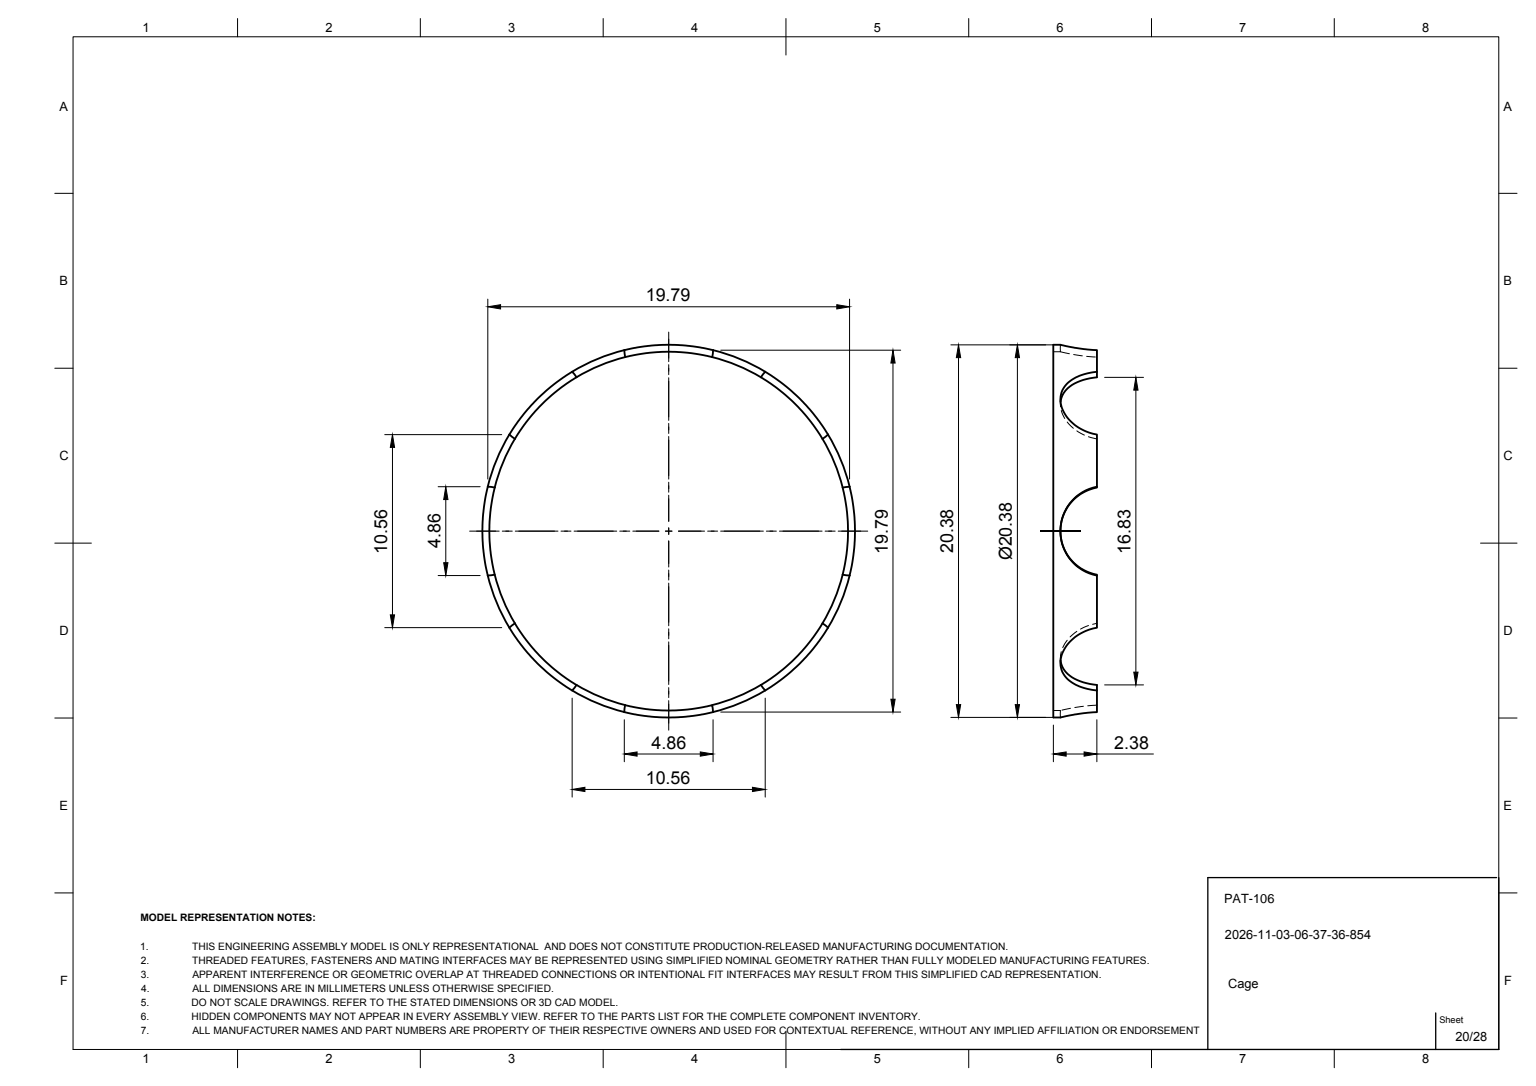
ISO-10303-21;
HEADER;
/* Generated by software containing ST-Developer
 * from STEP Tools, Inc. (www.steptools.com) 
 */

FILE_DESCRIPTION(
/* description */ ('Torsion-spring ratchet demonstrator'),
/* implementation_level */ '2;1');

FILE_NAME(
/* name */ 'Cage.step',
/* time_stamp */ '2026-10-29T17:29:17-07:00',
/* author */ (''),
/* organization */ (''),
/* preprocessor_version */ 'ST-DEVELOPER v20.2',
/* originating_system */ 'Autodesk Translation Framework v15.17.0.0',
/* authorisation */ '');

FILE_SCHEMA (('AUTOMOTIVE_DESIGN { 1 0 10303 214 3 1 1 }'));
ENDSEC;

DATA;
#10=MECHANICAL_DESIGN_GEOMETRIC_PRESENTATION_REPRESENTATION('',(#302),#11258);
#178=SPHERICAL_SURFACE('',#5739,0.247676);
#179=SPHERICAL_SURFACE('',#5755,0.247676);
#180=SPHERICAL_SURFACE('',#5760,0.247676);
#181=SPHERICAL_SURFACE('',#5765,0.247676);
#182=SPHERICAL_SURFACE('',#5770,0.247676);
#183=SPHERICAL_SURFACE('',#5775,0.247676);
#184=SPHERICAL_SURFACE('',#5780,0.247676);
#185=SPHERICAL_SURFACE('',#5788,0.247676);
#205=B_SPLINE_CURVE_WITH_KNOTS('',3,(#8316,#8317,#8318,#8319,#8320,#8321,
#8322,#8323,#8324,#8325,#8326,#8327,#8328,#8329,#8330,#8331,#8332,#8333,
#8334,#8335,#8336,#8337),.UNSPECIFIED.,.F.,.F.,(4,2,2,2,2,2,2,2,2,2,4),
(0.0473477652366656,0.126350602536658,0.189525903804987,0.252701205073317,
0.313298422430275,0.373895639787233,0.434492857144191,0.495090074501149,
0.558265375769478,0.621440677037807,0.7004435143378),.UNSPECIFIED.);
#206=B_SPLINE_CURVE_WITH_KNOTS('',3,(#8341,#8342,#8343,#8344,#8345,#8346,
#8347,#8348,#8349,#8350,#8351,#8352,#8353,#8354,#8355,#8356,#8357,#8358,
#8359,#8360,#8361,#8362),.UNSPECIFIED.,.F.,.F.,(4,2,2,2,2,2,2,2,2,2,4),
(0.0464897534940957,0.0852567806515119,0.170513561303024,0.246687263103517,
0.308657850341199,0.370628437578881,0.432599024816563,0.494569612054245,
0.570743313854739,0.656000094506251,0.694767121663666),.UNSPECIFIED.);
#207=B_SPLINE_CURVE_WITH_KNOTS('',3,(#8368,#8369,#8370,#8371,#8372,#8373,
#8374,#8375,#8376,#8377,#8378,#8379,#8380,#8381,#8382,#8383,#8384,#8385,
#8386,#8387,#8388,#8389),.UNSPECIFIED.,.F.,.F.,(4,2,2,2,2,2,2,2,2,2,4),
(0.0464897534940957,0.0852567806515118,0.170513561303024,0.246687263103517,
0.308657850341199,0.370628437578881,0.432599024816563,0.494569612054245,
0.570743313854738,0.65600009450625,0.694767121663666),.UNSPECIFIED.);
#208=B_SPLINE_CURVE_WITH_KNOTS('',3,(#8393,#8394,#8395,#8396,#8397,#8398,
#8399,#8400,#8401,#8402,#8403,#8404,#8405,#8406,#8407,#8408,#8409,#8410,
#8411,#8412,#8413,#8414),.UNSPECIFIED.,.F.,.F.,(4,2,2,2,2,2,2,2,2,2,4),
(0.0464897534940957,0.0852567806515119,0.170513561303024,0.246687263103517,
0.308657850341199,0.370628437578881,0.432599024816563,0.494569612054245,
0.570743313854739,0.656000094506251,0.694767121663666),.UNSPECIFIED.);
#209=B_SPLINE_CURVE_WITH_KNOTS('',3,(#8418,#8419,#8420,#8421,#8422,#8423,
#8424,#8425,#8426,#8427,#8428,#8429),.UNSPECIFIED.,.F.,.F.,(4,2,2,2,2,4),
(0.0464897534940957,0.0852567806515119,0.170513561303024,0.246687263103517,
0.308657850341199,0.370628437578881),.UNSPECIFIED.);
#210=B_SPLINE_CURVE_WITH_KNOTS('',3,(#8434,#8435,#8436,#8437,#8438,#8439,
#8440,#8441,#8442,#8443,#8444,#8445),.UNSPECIFIED.,.F.,.F.,(4,2,2,2,2,4),
(0.370628437578881,0.432599024816563,0.494569612054245,0.570743313854738,
0.65600009450625,0.694767121663666),.UNSPECIFIED.);
#211=B_SPLINE_CURVE_WITH_KNOTS('',3,(#8449,#8450,#8451,#8452,#8453,#8454,
#8455,#8456,#8457,#8458,#8459,#8460,#8461,#8462,#8463,#8464,#8465,#8466,
#8467,#8468,#8469,#8470),.UNSPECIFIED.,.F.,.F.,(4,2,2,2,2,2,2,2,2,2,4),
(0.0464897534940957,0.0852567806515121,0.170513561303024,0.246687263103518,
0.308657850341199,0.370628437578881,0.432599024816563,0.494569612054245,
0.570743313854738,0.65600009450625,0.694767121663666),.UNSPECIFIED.);
#212=B_SPLINE_CURVE_WITH_KNOTS('',3,(#8474,#8475,#8476,#8477,#8478,#8479,
#8480,#8481,#8482,#8483,#8484,#8485,#8486,#8487,#8488,#8489,#8490,#8491,
#8492,#8493,#8494,#8495),.UNSPECIFIED.,.F.,.F.,(4,2,2,2,2,2,2,2,2,2,4),
(0.0464897534940957,0.0852567806515119,0.170513561303024,0.246687263103517,
0.308657850341199,0.370628437578881,0.432599024816563,0.494569612054245,
0.570743313854738,0.65600009450625,0.694767121663667),.UNSPECIFIED.);
#213=B_SPLINE_CURVE_WITH_KNOTS('',3,(#8499,#8500,#8501,#8502,#8503,#8504,
#8505,#8506,#8507,#8508,#8509,#8510,#8511,#8512,#8513,#8514,#8515,#8516,
#8517,#8518,#8519,#8520),.UNSPECIFIED.,.F.,.F.,(4,2,2,2,2,2,2,2,2,2,4),
(0.0464897534940957,0.0852567806515119,0.170513561303024,0.246687263103517,
0.308657850341199,0.370628437578881,0.432599024816563,0.494569612054245,
0.570743313854738,0.65600009450625,0.694767121663666),.UNSPECIFIED.);
#214=B_SPLINE_CURVE_WITH_KNOTS('',3,(#8524,#8525,#8526,#8527,#8528,#8529,
#8530,#8531,#8532,#8533,#8534,#8535,#8536,#8537,#8538,#8539,#8540,#8541,
#8542,#8543,#8544,#8545),.UNSPECIFIED.,.F.,.F.,(4,2,2,2,2,2,2,2,2,2,4),
(0.0464897534940957,0.0852567806515119,0.170513561303024,0.246687263103517,
0.308657850341199,0.370628437578881,0.432599024816563,0.494569612054245,
0.570743313854739,0.656000094506251,0.694767121663667),.UNSPECIFIED.);
#215=B_SPLINE_CURVE_WITH_KNOTS('',3,(#8553,#8554,#8555,#8556,#8557,#8558,
#8559,#8560,#8561,#8562,#8563,#8564,#8565,#8566,#8567,#8568,#8569,#8570,
#8571,#8572,#8573,#8574),.UNSPECIFIED.,.F.,.F.,(4,2,2,2,2,2,2,2,2,2,4),
(0.0473477652366656,0.126350602536658,0.189525903804987,0.252701205073316,
0.313298422430274,0.373895639787232,0.434492857144191,0.495090074501149,
0.558265375769478,0.621440677037807,0.7004435143378),.UNSPECIFIED.);
#216=B_SPLINE_CURVE_WITH_KNOTS('',3,(#8582,#8583,#8584,#8585,#8586,#8587,
#8588,#8589,#8590,#8591,#8592,#8593,#8594,#8595,#8596,#8597,#8598,#8599,
#8600,#8601,#8602,#8603),.UNSPECIFIED.,.F.,.F.,(4,2,2,2,2,2,2,2,2,2,4),
(0.0473477652366656,0.126350602536658,0.189525903804987,0.252701205073317,
0.313298422430275,0.373895639787233,0.434492857144191,0.495090074501149,
0.558265375769478,0.621440677037807,0.7004435143378),.UNSPECIFIED.);
#217=B_SPLINE_CURVE_WITH_KNOTS('',3,(#8612,#8613,#8614,#8615,#8616,#8617,
#8618,#8619,#8620,#8621,#8622,#8623),.UNSPECIFIED.,.F.,.F.,(4,2,2,2,2,4),
(0.0473477652366656,0.126350602536658,0.189525903804987,0.252701205073316,
0.313298422430275,0.373895639787233),.UNSPECIFIED.);
#218=B_SPLINE_CURVE_WITH_KNOTS('',3,(#8625,#8626,#8627,#8628,#8629,#8630,
#8631,#8632,#8633,#8634,#8635,#8636),.UNSPECIFIED.,.F.,.F.,(4,2,2,2,2,4),
(0.373895639787233,0.434492857144191,0.495090074501149,0.558265375769478,
0.621440677037807,0.7004435143378),.UNSPECIFIED.);
#219=B_SPLINE_CURVE_WITH_KNOTS('',3,(#8643,#8644,#8645,#8646,#8647,#8648,
#8649,#8650,#8651,#8652,#8653,#8654,#8655,#8656,#8657,#8658,#8659,#8660,
#8661,#8662,#8663,#8664),.UNSPECIFIED.,.F.,.F.,(4,2,2,2,2,2,2,2,2,2,4),
(0.0473477652366656,0.126350602536658,0.189525903804987,0.252701205073316,
0.313298422430275,0.373895639787233,0.434492857144191,0.495090074501149,
0.558265375769478,0.621440677037807,0.7004435143378),.UNSPECIFIED.);
#220=B_SPLINE_CURVE_WITH_KNOTS('',3,(#8672,#8673,#8674,#8675,#8676,#8677,
#8678,#8679,#8680,#8681,#8682,#8683,#8684,#8685,#8686,#8687,#8688,#8689,
#8690,#8691,#8692,#8693),.UNSPECIFIED.,.F.,.F.,(4,2,2,2,2,2,2,2,2,2,4),
(0.0473477652366656,0.126350602536658,0.189525903804987,0.252701205073317,
0.313298422430275,0.373895639787233,0.434492857144191,0.495090074501149,
0.558265375769478,0.621440677037807,0.7004435143378),.UNSPECIFIED.);
#221=B_SPLINE_CURVE_WITH_KNOTS('',3,(#8701,#8702,#8703,#8704,#8705,#8706,
#8707,#8708,#8709,#8710,#8711,#8712,#8713,#8714,#8715,#8716,#8717,#8718,
#8719,#8720,#8721,#8722),.UNSPECIFIED.,.F.,.F.,(4,2,2,2,2,2,2,2,2,2,4),
(0.0473477652366656,0.126350602536658,0.189525903804987,0.252701205073316,
0.313298422430275,0.373895639787233,0.434492857144191,0.495090074501149,
0.558265375769478,0.621440677037807,0.7004435143378),.UNSPECIFIED.);
#222=B_SPLINE_CURVE_WITH_KNOTS('',3,(#8731,#8732,#8733,#8734,#8735,#8736,
#8737,#8738,#8739,#8740,#8741,#8742,#8743,#8744,#8745,#8746,#8747,#8748,
#8749,#8750,#8751,#8752),.UNSPECIFIED.,.F.,.F.,(4,2,2,2,2,2,2,2,2,2,4),
(0.0473477652366656,0.126350602536658,0.189525903804987,0.252701205073317,
0.313298422430275,0.373895639787233,0.434492857144191,0.495090074501149,
0.558265375769478,0.621440677037807,0.7004435143378),.UNSPECIFIED.);
#247=SHAPE_REPRESENTATION_RELATIONSHIP('SRR','None',#11374,#271);
#271=ADVANCED_BREP_SHAPE_REPRESENTATION('',(#334),#11244);
#302=STYLED_ITEM('',(#11584),#334);
#334=MANIFOLD_SOLID_BREP('Continuous crown cage',#5173);
#413=FACE_BOUND('',#1142,.T.);
#493=PLANE('',#5752);
#494=PLANE('',#5757);
#495=PLANE('',#5762);
#496=PLANE('',#5767);
#497=PLANE('',#5772);
#498=PLANE('',#5777);
#499=PLANE('',#5786);
#500=PLANE('',#5790);
#501=PLANE('',#5791);
#751=FACE_OUTER_BOUND('',#1124,.T.);
#752=FACE_OUTER_BOUND('',#1125,.T.);
#753=FACE_OUTER_BOUND('',#1126,.T.);
#754=FACE_OUTER_BOUND('',#1127,.T.);
#755=FACE_OUTER_BOUND('',#1128,.T.);
#756=FACE_OUTER_BOUND('',#1129,.T.);
#757=FACE_OUTER_BOUND('',#1130,.T.);
#758=FACE_OUTER_BOUND('',#1131,.T.);
#759=FACE_OUTER_BOUND('',#1132,.T.);
#760=FACE_OUTER_BOUND('',#1133,.T.);
#761=FACE_OUTER_BOUND('',#1134,.T.);
#762=FACE_OUTER_BOUND('',#1135,.T.);
#763=FACE_OUTER_BOUND('',#1136,.T.);
#764=FACE_OUTER_BOUND('',#1137,.T.);
#765=FACE_OUTER_BOUND('',#1138,.T.);
#766=FACE_OUTER_BOUND('',#1139,.T.);
#767=FACE_OUTER_BOUND('',#1140,.T.);
#768=FACE_OUTER_BOUND('',#1141,.T.);
#769=FACE_OUTER_BOUND('',#1143,.T.);
#1124=EDGE_LOOP('',(#3942,#3943,#3944,#3945));
#1125=EDGE_LOOP('',(#3946,#3947,#3948,#3949,#3950,#3951,#3952,#3953,#3954,
#3955,#3956,#3957,#3958,#3959,#3960,#3961,#3962,#3963,#3964,#3965));
#1126=EDGE_LOOP('',(#3966,#3967,#3968,#3969));
#1127=EDGE_LOOP('',(#3970,#3971,#3972,#3973));
#1128=EDGE_LOOP('',(#3974,#3975,#3976,#3977));
#1129=EDGE_LOOP('',(#3978,#3979,#3980,#3981));
#1130=EDGE_LOOP('',(#3982,#3983,#3984,#3985));
#1131=EDGE_LOOP('',(#3986,#3987,#3988,#3989,#3990,#3991));
#1132=EDGE_LOOP('',(#3992,#3993,#3994,#3995));
#1133=EDGE_LOOP('',(#3996,#3997,#3998,#3999));
#1134=EDGE_LOOP('',(#4000,#4001,#4002,#4003));
#1135=EDGE_LOOP('',(#4004,#4005,#4006,#4007));
#1136=EDGE_LOOP('',(#4008,#4009,#4010,#4011));
#1137=EDGE_LOOP('',(#4012,#4013,#4014,#4015));
#1138=EDGE_LOOP('',(#4016,#4017,#4018,#4019,#4020,#4021,#4022,#4023,#4024,
#4025,#4026,#4027,#4028,#4029,#4030,#4031,#4032,#4033,#4034,#4035));
#1139=EDGE_LOOP('',(#4036,#4037,#4038,#4039));
#1140=EDGE_LOOP('',(#4040,#4041,#4042,#4043));
#1141=EDGE_LOOP('',(#4044));
#1142=EDGE_LOOP('',(#4045));
#1143=EDGE_LOOP('',(#4046,#4047,#4048,#4049));
#1429=LINE('',#8431,#1812);
#1430=LINE('',#8727,#1813);
#1812=VECTOR('',#6756,1.019052);
#1813=VECTOR('',#6833,0.980948);
#2233=CIRCLE('',#5740,0.243053047864041);
#2234=CIRCLE('',#5741,0.243053047864041);
#2235=CIRCLE('',#5743,1.019052);
#2236=CIRCLE('',#5744,1.019052);
#2237=CIRCLE('',#5745,1.019052);
#2238=CIRCLE('',#5746,1.019052);
#2239=CIRCLE('',#5747,1.019052);
#2240=CIRCLE('',#5748,1.019052);
#2241=CIRCLE('',#5749,1.019052);
#2242=CIRCLE('',#5750,1.019052);
#2243=CIRCLE('',#5751,1.019052);
#2244=CIRCLE('',#5753,0.980948);
#2245=CIRCLE('',#5754,0.243053047864041);
#2246=CIRCLE('',#5756,0.243053047864041);
#2247=CIRCLE('',#5758,0.980948);
#2248=CIRCLE('',#5759,0.243053047864041);
#2249=CIRCLE('',#5761,0.243053047864041);
#2250=CIRCLE('',#5763,0.980948);
#2251=CIRCLE('',#5764,0.243053047864041);
#2252=CIRCLE('',#5766,0.243053047864041);
#2253=CIRCLE('',#5768,0.980948);
#2254=CIRCLE('',#5769,0.243053047864041);
#2255=CIRCLE('',#5771,0.243053047864041);
#2256=CIRCLE('',#5773,0.980948);
#2257=CIRCLE('',#5774,0.243053047864041);
#2258=CIRCLE('',#5776,0.243053047864041);
#2259=CIRCLE('',#5778,0.980948);
#2260=CIRCLE('',#5779,0.243053047864041);
#2261=CIRCLE('',#5781,0.243053047864041);
#2262=CIRCLE('',#5783,0.980948);
#2263=CIRCLE('',#5784,0.980948);
#2264=CIRCLE('',#5785,0.980948);
#2265=CIRCLE('',#5787,0.243053047864041);
#2266=CIRCLE('',#5789,0.243053047864041);
#2511=VERTEX_POINT('',#8314);
#2512=VERTEX_POINT('',#8315);
#2513=VERTEX_POINT('',#8338);
#2514=VERTEX_POINT('',#8340);
#2515=VERTEX_POINT('',#8365);
#2516=VERTEX_POINT('',#8367);
#2517=VERTEX_POINT('',#8390);
#2518=VERTEX_POINT('',#8392);
#2519=VERTEX_POINT('',#8415);
#2520=VERTEX_POINT('',#8417);
#2521=VERTEX_POINT('',#8430);
#2522=VERTEX_POINT('',#8433);
#2523=VERTEX_POINT('',#8446);
#2524=VERTEX_POINT('',#8448);
#2525=VERTEX_POINT('',#8471);
#2526=VERTEX_POINT('',#8473);
#2527=VERTEX_POINT('',#8496);
#2528=VERTEX_POINT('',#8498);
#2529=VERTEX_POINT('',#8521);
#2530=VERTEX_POINT('',#8523);
#2531=VERTEX_POINT('',#8548);
#2532=VERTEX_POINT('',#8552);
#2533=VERTEX_POINT('',#8577);
#2534=VERTEX_POINT('',#8581);
#2535=VERTEX_POINT('',#8606);
#2536=VERTEX_POINT('',#8610);
#2537=VERTEX_POINT('',#8611);
#2538=VERTEX_POINT('',#8638);
#2539=VERTEX_POINT('',#8642);
#2540=VERTEX_POINT('',#8667);
#2541=VERTEX_POINT('',#8671);
#2542=VERTEX_POINT('',#8696);
#2543=VERTEX_POINT('',#8700);
#2544=VERTEX_POINT('',#8725);
#2545=VERTEX_POINT('',#8728);
#2546=VERTEX_POINT('',#8730);
#3031=EDGE_CURVE('',#2511,#2512,#205,.T.);
#3032=EDGE_CURVE('',#2513,#2511,#2233,.T.);
#3033=EDGE_CURVE('',#2514,#2513,#206,.T.);
#3034=EDGE_CURVE('',#2512,#2514,#2234,.T.);
#3035=EDGE_CURVE('',#2515,#2513,#2235,.T.);
#3036=EDGE_CURVE('',#2515,#2516,#207,.T.);
#3037=EDGE_CURVE('',#2517,#2516,#2236,.T.);
#3038=EDGE_CURVE('',#2517,#2518,#208,.T.);
#3039=EDGE_CURVE('',#2519,#2518,#2237,.T.);
#3040=EDGE_CURVE('',#2519,#2520,#209,.T.);
#3041=EDGE_CURVE('',#2520,#2521,#1429,.T.);
#3042=EDGE_CURVE('',#2521,#2521,#2238,.T.);
#3043=EDGE_CURVE('',#2520,#2522,#210,.T.);
#3044=EDGE_CURVE('',#2523,#2522,#2239,.T.);
#3045=EDGE_CURVE('',#2523,#2524,#211,.T.);
#3046=EDGE_CURVE('',#2525,#2524,#2240,.T.);
#3047=EDGE_CURVE('',#2525,#2526,#212,.T.);
#3048=EDGE_CURVE('',#2527,#2526,#2241,.T.);
#3049=EDGE_CURVE('',#2527,#2528,#213,.T.);
#3050=EDGE_CURVE('',#2529,#2528,#2242,.T.);
#3051=EDGE_CURVE('',#2529,#2530,#214,.T.);
#3052=EDGE_CURVE('',#2514,#2530,#2243,.T.);
#3053=EDGE_CURVE('',#2511,#2531,#2244,.T.);
#3054=EDGE_CURVE('',#2531,#2515,#2245,.T.);
#3055=EDGE_CURVE('',#2532,#2531,#215,.T.);
#3056=EDGE_CURVE('',#2516,#2532,#2246,.T.);
#3057=EDGE_CURVE('',#2532,#2533,#2247,.T.);
#3058=EDGE_CURVE('',#2533,#2517,#2248,.T.);
#3059=EDGE_CURVE('',#2534,#2533,#216,.T.);
#3060=EDGE_CURVE('',#2518,#2534,#2249,.T.);
#3061=EDGE_CURVE('',#2534,#2535,#2250,.T.);
#3062=EDGE_CURVE('',#2535,#2519,#2251,.T.);
#3063=EDGE_CURVE('',#2536,#2537,#217,.T.);
#3064=EDGE_CURVE('',#2522,#2536,#2252,.T.);
#3065=EDGE_CURVE('',#2537,#2535,#218,.T.);
#3066=EDGE_CURVE('',#2536,#2538,#2253,.T.);
#3067=EDGE_CURVE('',#2538,#2523,#2254,.T.);
#3068=EDGE_CURVE('',#2539,#2538,#219,.T.);
#3069=EDGE_CURVE('',#2524,#2539,#2255,.T.);
#3070=EDGE_CURVE('',#2539,#2540,#2256,.T.);
#3071=EDGE_CURVE('',#2540,#2525,#2257,.T.);
#3072=EDGE_CURVE('',#2541,#2540,#220,.T.);
#3073=EDGE_CURVE('',#2526,#2541,#2258,.T.);
#3074=EDGE_CURVE('',#2541,#2542,#2259,.T.);
#3075=EDGE_CURVE('',#2542,#2527,#2260,.T.);
#3076=EDGE_CURVE('',#2543,#2542,#221,.T.);
#3077=EDGE_CURVE('',#2528,#2543,#2261,.T.);
#3078=EDGE_CURVE('',#2544,#2544,#2262,.T.);
#3079=EDGE_CURVE('',#2544,#2537,#1430,.T.);
#3080=EDGE_CURVE('',#2545,#2512,#2263,.T.);
#3081=EDGE_CURVE('',#2545,#2546,#222,.T.);
#3082=EDGE_CURVE('',#2543,#2546,#2264,.T.);
#3083=EDGE_CURVE('',#2530,#2545,#2265,.T.);
#3084=EDGE_CURVE('',#2546,#2529,#2266,.T.);
#3942=ORIENTED_EDGE('',*,*,#3031,.F.);
#3943=ORIENTED_EDGE('',*,*,#3032,.F.);
#3944=ORIENTED_EDGE('',*,*,#3033,.F.);
#3945=ORIENTED_EDGE('',*,*,#3034,.F.);
#3946=ORIENTED_EDGE('',*,*,#3033,.T.);
#3947=ORIENTED_EDGE('',*,*,#3035,.F.);
#3948=ORIENTED_EDGE('',*,*,#3036,.T.);
#3949=ORIENTED_EDGE('',*,*,#3037,.F.);
#3950=ORIENTED_EDGE('',*,*,#3038,.T.);
#3951=ORIENTED_EDGE('',*,*,#3039,.F.);
#3952=ORIENTED_EDGE('',*,*,#3040,.T.);
#3953=ORIENTED_EDGE('',*,*,#3041,.T.);
#3954=ORIENTED_EDGE('',*,*,#3042,.F.);
#3955=ORIENTED_EDGE('',*,*,#3041,.F.);
#3956=ORIENTED_EDGE('',*,*,#3043,.T.);
#3957=ORIENTED_EDGE('',*,*,#3044,.F.);
#3958=ORIENTED_EDGE('',*,*,#3045,.T.);
#3959=ORIENTED_EDGE('',*,*,#3046,.F.);
#3960=ORIENTED_EDGE('',*,*,#3047,.T.);
#3961=ORIENTED_EDGE('',*,*,#3048,.F.);
#3962=ORIENTED_EDGE('',*,*,#3049,.T.);
#3963=ORIENTED_EDGE('',*,*,#3050,.F.);
#3964=ORIENTED_EDGE('',*,*,#3051,.T.);
#3965=ORIENTED_EDGE('',*,*,#3052,.F.);
#3966=ORIENTED_EDGE('',*,*,#3032,.T.);
#3967=ORIENTED_EDGE('',*,*,#3053,.T.);
#3968=ORIENTED_EDGE('',*,*,#3054,.T.);
#3969=ORIENTED_EDGE('',*,*,#3035,.T.);
#3970=ORIENTED_EDGE('',*,*,#3055,.F.);
#3971=ORIENTED_EDGE('',*,*,#3056,.F.);
#3972=ORIENTED_EDGE('',*,*,#3036,.F.);
#3973=ORIENTED_EDGE('',*,*,#3054,.F.);
#3974=ORIENTED_EDGE('',*,*,#3056,.T.);
#3975=ORIENTED_EDGE('',*,*,#3057,.T.);
#3976=ORIENTED_EDGE('',*,*,#3058,.T.);
#3977=ORIENTED_EDGE('',*,*,#3037,.T.);
#3978=ORIENTED_EDGE('',*,*,#3059,.F.);
#3979=ORIENTED_EDGE('',*,*,#3060,.F.);
#3980=ORIENTED_EDGE('',*,*,#3038,.F.);
#3981=ORIENTED_EDGE('',*,*,#3058,.F.);
#3982=ORIENTED_EDGE('',*,*,#3060,.T.);
#3983=ORIENTED_EDGE('',*,*,#3061,.T.);
#3984=ORIENTED_EDGE('',*,*,#3062,.T.);
#3985=ORIENTED_EDGE('',*,*,#3039,.T.);
#3986=ORIENTED_EDGE('',*,*,#3063,.F.);
#3987=ORIENTED_EDGE('',*,*,#3064,.F.);
#3988=ORIENTED_EDGE('',*,*,#3043,.F.);
#3989=ORIENTED_EDGE('',*,*,#3040,.F.);
#3990=ORIENTED_EDGE('',*,*,#3062,.F.);
#3991=ORIENTED_EDGE('',*,*,#3065,.F.);
#3992=ORIENTED_EDGE('',*,*,#3064,.T.);
#3993=ORIENTED_EDGE('',*,*,#3066,.T.);
#3994=ORIENTED_EDGE('',*,*,#3067,.T.);
#3995=ORIENTED_EDGE('',*,*,#3044,.T.);
#3996=ORIENTED_EDGE('',*,*,#3068,.F.);
#3997=ORIENTED_EDGE('',*,*,#3069,.F.);
#3998=ORIENTED_EDGE('',*,*,#3045,.F.);
#3999=ORIENTED_EDGE('',*,*,#3067,.F.);
#4000=ORIENTED_EDGE('',*,*,#3069,.T.);
#4001=ORIENTED_EDGE('',*,*,#3070,.T.);
#4002=ORIENTED_EDGE('',*,*,#3071,.T.);
#4003=ORIENTED_EDGE('',*,*,#3046,.T.);
#4004=ORIENTED_EDGE('',*,*,#3072,.F.);
#4005=ORIENTED_EDGE('',*,*,#3073,.F.);
#4006=ORIENTED_EDGE('',*,*,#3047,.F.);
#4007=ORIENTED_EDGE('',*,*,#3071,.F.);
#4008=ORIENTED_EDGE('',*,*,#3073,.T.);
#4009=ORIENTED_EDGE('',*,*,#3074,.T.);
#4010=ORIENTED_EDGE('',*,*,#3075,.T.);
#4011=ORIENTED_EDGE('',*,*,#3048,.T.);
#4012=ORIENTED_EDGE('',*,*,#3049,.F.);
#4013=ORIENTED_EDGE('',*,*,#3075,.F.);
#4014=ORIENTED_EDGE('',*,*,#3076,.F.);
#4015=ORIENTED_EDGE('',*,*,#3077,.F.);
#4016=ORIENTED_EDGE('',*,*,#3078,.F.);
#4017=ORIENTED_EDGE('',*,*,#3079,.T.);
#4018=ORIENTED_EDGE('',*,*,#3065,.T.);
#4019=ORIENTED_EDGE('',*,*,#3061,.F.);
#4020=ORIENTED_EDGE('',*,*,#3059,.T.);
#4021=ORIENTED_EDGE('',*,*,#3057,.F.);
#4022=ORIENTED_EDGE('',*,*,#3055,.T.);
#4023=ORIENTED_EDGE('',*,*,#3053,.F.);
#4024=ORIENTED_EDGE('',*,*,#3031,.T.);
#4025=ORIENTED_EDGE('',*,*,#3080,.F.);
#4026=ORIENTED_EDGE('',*,*,#3081,.T.);
#4027=ORIENTED_EDGE('',*,*,#3082,.F.);
#4028=ORIENTED_EDGE('',*,*,#3076,.T.);
#4029=ORIENTED_EDGE('',*,*,#3074,.F.);
#4030=ORIENTED_EDGE('',*,*,#3072,.T.);
#4031=ORIENTED_EDGE('',*,*,#3070,.F.);
#4032=ORIENTED_EDGE('',*,*,#3068,.T.);
#4033=ORIENTED_EDGE('',*,*,#3066,.F.);
#4034=ORIENTED_EDGE('',*,*,#3063,.T.);
#4035=ORIENTED_EDGE('',*,*,#3079,.F.);
#4036=ORIENTED_EDGE('',*,*,#3034,.T.);
#4037=ORIENTED_EDGE('',*,*,#3052,.T.);
#4038=ORIENTED_EDGE('',*,*,#3083,.T.);
#4039=ORIENTED_EDGE('',*,*,#3080,.T.);
#4040=ORIENTED_EDGE('',*,*,#3051,.F.);
#4041=ORIENTED_EDGE('',*,*,#3084,.F.);
#4042=ORIENTED_EDGE('',*,*,#3081,.F.);
#4043=ORIENTED_EDGE('',*,*,#3083,.F.);
#4044=ORIENTED_EDGE('',*,*,#3042,.T.);
#4045=ORIENTED_EDGE('',*,*,#3078,.T.);
#4046=ORIENTED_EDGE('',*,*,#3077,.T.);
#4047=ORIENTED_EDGE('',*,*,#3082,.T.);
#4048=ORIENTED_EDGE('',*,*,#3084,.T.);
#4049=ORIENTED_EDGE('',*,*,#3050,.T.);
#4822=CYLINDRICAL_SURFACE('',#5742,1.019052);
#4823=CYLINDRICAL_SURFACE('',#5782,0.980948);
#4977=ADVANCED_FACE('',(#751),#178,.F.);
#4978=ADVANCED_FACE('',(#752),#4822,.T.);
#4979=ADVANCED_FACE('',(#753),#493,.T.);
#4980=ADVANCED_FACE('',(#754),#179,.F.);
#4981=ADVANCED_FACE('',(#755),#494,.T.);
#4982=ADVANCED_FACE('',(#756),#180,.F.);
#4983=ADVANCED_FACE('',(#757),#495,.T.);
#4984=ADVANCED_FACE('',(#758),#181,.F.);
#4985=ADVANCED_FACE('',(#759),#496,.T.);
#4986=ADVANCED_FACE('',(#760),#182,.F.);
#4987=ADVANCED_FACE('',(#761),#497,.T.);
#4988=ADVANCED_FACE('',(#762),#183,.F.);
#4989=ADVANCED_FACE('',(#763),#498,.T.);
#4990=ADVANCED_FACE('',(#764),#184,.F.);
#4991=ADVANCED_FACE('',(#765),#4823,.F.);
#4992=ADVANCED_FACE('',(#766),#499,.T.);
#4993=ADVANCED_FACE('',(#767),#185,.F.);
#4994=ADVANCED_FACE('',(#768,#413),#500,.T.);
#4995=ADVANCED_FACE('',(#769),#501,.T.);
#5173=CLOSED_SHELL('',(#4977,#4978,#4979,#4980,#4981,#4982,#4983,#4984,
#4985,#4986,#4987,#4988,#4989,#4990,#4991,#4992,#4993,#4994,#4995));
#5738=AXIS2_PLACEMENT_3D('',#8312,#6740,#6741);
#5739=AXIS2_PLACEMENT_3D('',#8313,#6742,#6743);
#5740=AXIS2_PLACEMENT_3D('',#8339,#6744,#6745);
#5741=AXIS2_PLACEMENT_3D('',#8363,#6746,#6747);
#5742=AXIS2_PLACEMENT_3D('',#8364,#6748,#6749);
#5743=AXIS2_PLACEMENT_3D('',#8366,#6750,#6751);
#5744=AXIS2_PLACEMENT_3D('',#8391,#6752,#6753);
#5745=AXIS2_PLACEMENT_3D('',#8416,#6754,#6755);
#5746=AXIS2_PLACEMENT_3D('',#8432,#6757,#6758);
#5747=AXIS2_PLACEMENT_3D('',#8447,#6759,#6760);
#5748=AXIS2_PLACEMENT_3D('',#8472,#6761,#6762);
#5749=AXIS2_PLACEMENT_3D('',#8497,#6763,#6764);
#5750=AXIS2_PLACEMENT_3D('',#8522,#6765,#6766);
#5751=AXIS2_PLACEMENT_3D('',#8546,#6767,#6768);
#5752=AXIS2_PLACEMENT_3D('',#8547,#6769,#6770);
#5753=AXIS2_PLACEMENT_3D('',#8549,#6771,#6772);
#5754=AXIS2_PLACEMENT_3D('',#8550,#6773,#6774);
#5755=AXIS2_PLACEMENT_3D('',#8551,#6775,#6776);
#5756=AXIS2_PLACEMENT_3D('',#8575,#6777,#6778);
#5757=AXIS2_PLACEMENT_3D('',#8576,#6779,#6780);
#5758=AXIS2_PLACEMENT_3D('',#8578,#6781,#6782);
#5759=AXIS2_PLACEMENT_3D('',#8579,#6783,#6784);
#5760=AXIS2_PLACEMENT_3D('',#8580,#6785,#6786);
#5761=AXIS2_PLACEMENT_3D('',#8604,#6787,#6788);
#5762=AXIS2_PLACEMENT_3D('',#8605,#6789,#6790);
#5763=AXIS2_PLACEMENT_3D('',#8607,#6791,#6792);
#5764=AXIS2_PLACEMENT_3D('',#8608,#6793,#6794);
#5765=AXIS2_PLACEMENT_3D('',#8609,#6795,#6796);
#5766=AXIS2_PLACEMENT_3D('',#8624,#6797,#6798);
#5767=AXIS2_PLACEMENT_3D('',#8637,#6799,#6800);
#5768=AXIS2_PLACEMENT_3D('',#8639,#6801,#6802);
#5769=AXIS2_PLACEMENT_3D('',#8640,#6803,#6804);
#5770=AXIS2_PLACEMENT_3D('',#8641,#6805,#6806);
#5771=AXIS2_PLACEMENT_3D('',#8665,#6807,#6808);
#5772=AXIS2_PLACEMENT_3D('',#8666,#6809,#6810);
#5773=AXIS2_PLACEMENT_3D('',#8668,#6811,#6812);
#5774=AXIS2_PLACEMENT_3D('',#8669,#6813,#6814);
#5775=AXIS2_PLACEMENT_3D('',#8670,#6815,#6816);
#5776=AXIS2_PLACEMENT_3D('',#8694,#6817,#6818);
#5777=AXIS2_PLACEMENT_3D('',#8695,#6819,#6820);
#5778=AXIS2_PLACEMENT_3D('',#8697,#6821,#6822);
#5779=AXIS2_PLACEMENT_3D('',#8698,#6823,#6824);
#5780=AXIS2_PLACEMENT_3D('',#8699,#6825,#6826);
#5781=AXIS2_PLACEMENT_3D('',#8723,#6827,#6828);
#5782=AXIS2_PLACEMENT_3D('',#8724,#6829,#6830);
#5783=AXIS2_PLACEMENT_3D('',#8726,#6831,#6832);
#5784=AXIS2_PLACEMENT_3D('',#8729,#6834,#6835);
#5785=AXIS2_PLACEMENT_3D('',#8753,#6836,#6837);
#5786=AXIS2_PLACEMENT_3D('',#8754,#6838,#6839);
#5787=AXIS2_PLACEMENT_3D('',#8755,#6840,#6841);
#5788=AXIS2_PLACEMENT_3D('',#8756,#6842,#6843);
#5789=AXIS2_PLACEMENT_3D('',#8757,#6844,#6845);
#5790=AXIS2_PLACEMENT_3D('',#8758,#6846,#6847);
#5791=AXIS2_PLACEMENT_3D('',#8759,#6848,#6849);
#6740=DIRECTION('axis',(0.,0.,1.));
#6741=DIRECTION('refdir',(1.,0.,0.));
#6742=DIRECTION('center_axis',(0.,0.,1.));
#6743=DIRECTION('ref_axis',(1.,0.,0.));
#6744=DIRECTION('center_axis',(0.,-1.,0.));
#6745=DIRECTION('ref_axis',(0.,0.,-1.));
#6746=DIRECTION('center_axis',(0.,-1.,0.));
#6747=DIRECTION('ref_axis',(0.,0.,-1.));
#6748=DIRECTION('center_axis',(0.,1.,0.));
#6749=DIRECTION('ref_axis',(1.,0.,0.));
#6750=DIRECTION('center_axis',(0.,1.,0.));
#6751=DIRECTION('ref_axis',(1.,0.,0.));
#6752=DIRECTION('center_axis',(0.,1.,0.));
#6753=DIRECTION('ref_axis',(1.,0.,0.));
#6754=DIRECTION('center_axis',(0.,1.,0.));
#6755=DIRECTION('ref_axis',(1.,0.,0.));
#6756=DIRECTION('',(0.,-1.,0.));
#6757=DIRECTION('center_axis',(0.,-1.,0.));
#6758=DIRECTION('ref_axis',(1.,0.,0.));
#6759=DIRECTION('center_axis',(0.,1.,0.));
#6760=DIRECTION('ref_axis',(1.,0.,0.));
#6761=DIRECTION('center_axis',(0.,1.,0.));
#6762=DIRECTION('ref_axis',(1.,0.,0.));
#6763=DIRECTION('center_axis',(0.,1.,0.));
#6764=DIRECTION('ref_axis',(1.,0.,0.));
#6765=DIRECTION('center_axis',(0.,1.,0.));
#6766=DIRECTION('ref_axis',(1.,0.,0.));
#6767=DIRECTION('center_axis',(0.,1.,0.));
#6768=DIRECTION('ref_axis',(1.,0.,0.));
#6769=DIRECTION('center_axis',(0.,1.,0.));
#6770=DIRECTION('ref_axis',(1.,0.,0.));
#6771=DIRECTION('center_axis',(0.,-1.,0.));
#6772=DIRECTION('ref_axis',(1.,0.,0.));
#6773=DIRECTION('center_axis',(0.,-1.,0.));
#6774=DIRECTION('ref_axis',(0.,0.,-1.));
#6775=DIRECTION('center_axis',(6.12323399573677E-17,0.,1.));
#6776=DIRECTION('ref_axis',(1.,0.,0.));
#6777=DIRECTION('center_axis',(0.,-1.,0.));
#6778=DIRECTION('ref_axis',(0.,0.,-1.));
#6779=DIRECTION('center_axis',(0.,1.,0.));
#6780=DIRECTION('ref_axis',(1.,0.,0.));
#6781=DIRECTION('center_axis',(0.,-1.,0.));
#6782=DIRECTION('ref_axis',(1.,0.,0.));
#6783=DIRECTION('center_axis',(0.,-1.,0.));
#6784=DIRECTION('ref_axis',(0.,0.,-1.));
#6785=DIRECTION('center_axis',(0.,0.,1.));
#6786=DIRECTION('ref_axis',(1.,0.,0.));
#6787=DIRECTION('center_axis',(0.,-1.,0.));
#6788=DIRECTION('ref_axis',(0.,0.,-1.));
#6789=DIRECTION('center_axis',(0.,1.,0.));
#6790=DIRECTION('ref_axis',(1.,0.,0.));
#6791=DIRECTION('center_axis',(0.,-1.,0.));
#6792=DIRECTION('ref_axis',(1.,0.,0.));
#6793=DIRECTION('center_axis',(0.,-1.,0.));
#6794=DIRECTION('ref_axis',(0.,0.,-1.));
#6795=DIRECTION('center_axis',(0.,0.,1.));
#6796=DIRECTION('ref_axis',(1.,0.,0.));
#6797=DIRECTION('center_axis',(0.,-1.,0.));
#6798=DIRECTION('ref_axis',(0.,0.,-1.));
#6799=DIRECTION('center_axis',(0.,1.,0.));
#6800=DIRECTION('ref_axis',(1.,0.,0.));
#6801=DIRECTION('center_axis',(0.,-1.,0.));
#6802=DIRECTION('ref_axis',(1.,0.,0.));
#6803=DIRECTION('center_axis',(0.,-1.,0.));
#6804=DIRECTION('ref_axis',(0.,0.,-1.));
#6805=DIRECTION('center_axis',(0.,0.,1.));
#6806=DIRECTION('ref_axis',(1.,0.,0.));
#6807=DIRECTION('center_axis',(0.,-1.,0.));
#6808=DIRECTION('ref_axis',(0.,0.,-1.));
#6809=DIRECTION('center_axis',(0.,1.,0.));
#6810=DIRECTION('ref_axis',(1.,0.,0.));
#6811=DIRECTION('center_axis',(0.,-1.,0.));
#6812=DIRECTION('ref_axis',(1.,0.,0.));
#6813=DIRECTION('center_axis',(0.,-1.,0.));
#6814=DIRECTION('ref_axis',(0.,0.,-1.));
#6815=DIRECTION('center_axis',(6.12323399573676E-17,0.,1.));
#6816=DIRECTION('ref_axis',(1.,0.,0.));
#6817=DIRECTION('center_axis',(0.,-1.,0.));
#6818=DIRECTION('ref_axis',(0.,0.,-1.));
#6819=DIRECTION('center_axis',(0.,1.,0.));
#6820=DIRECTION('ref_axis',(1.,0.,0.));
#6821=DIRECTION('center_axis',(0.,-1.,0.));
#6822=DIRECTION('ref_axis',(1.,0.,0.));
#6823=DIRECTION('center_axis',(0.,-1.,0.));
#6824=DIRECTION('ref_axis',(0.,0.,-1.));
#6825=DIRECTION('center_axis',(0.,0.,1.));
#6826=DIRECTION('ref_axis',(1.,0.,0.));
#6827=DIRECTION('center_axis',(0.,-1.,0.));
#6828=DIRECTION('ref_axis',(0.,0.,-1.));
#6829=DIRECTION('center_axis',(0.,1.,0.));
#6830=DIRECTION('ref_axis',(1.,0.,0.));
#6831=DIRECTION('center_axis',(0.,1.,0.));
#6832=DIRECTION('ref_axis',(1.,0.,0.));
#6833=DIRECTION('',(0.,1.,0.));
#6834=DIRECTION('center_axis',(0.,-1.,0.));
#6835=DIRECTION('ref_axis',(1.,0.,0.));
#6836=DIRECTION('center_axis',(0.,-1.,0.));
#6837=DIRECTION('ref_axis',(1.,0.,0.));
#6838=DIRECTION('center_axis',(0.,1.,0.));
#6839=DIRECTION('ref_axis',(1.,0.,0.));
#6840=DIRECTION('center_axis',(0.,-1.,0.));
#6841=DIRECTION('ref_axis',(0.,0.,-1.));
#6842=DIRECTION('center_axis',(0.,0.,1.));
#6843=DIRECTION('ref_axis',(1.,0.,0.));
#6844=DIRECTION('center_axis',(0.,-1.,0.));
#6845=DIRECTION('ref_axis',(0.,0.,-1.));
#6846=DIRECTION('center_axis',(0.,-1.,0.));
#6847=DIRECTION('ref_axis',(-1.,0.,0.));
#6848=DIRECTION('center_axis',(0.,1.,0.));
#6849=DIRECTION('ref_axis',(1.,0.,0.));
#8312=CARTESIAN_POINT('',(0.,0.,0.));
#8313=CARTESIAN_POINT('Origin',(0.707106781186547,0.,0.707106781186548));
#8314=CARTESIAN_POINT('',(0.504455939115715,-0.04763,0.841298510752802));
#8315=CARTESIAN_POINT('',(0.841298510752802,-0.04763,0.504455939115715));
#8316=CARTESIAN_POINT('Ctrl Pts',(0.504455939115715,-0.04763,0.841298510752802));
#8317=CARTESIAN_POINT('Ctrl Pts',(0.508899795931835,-0.0740444353928835,
0.838633903678357));
#8318=CARTESIAN_POINT('Ctrl Pts',(0.517157748491652,-0.0999305678883309,
0.833661031856294));
#8319=CARTESIAN_POINT('Ctrl Pts',(0.537715343527944,-0.142345102874864,
0.820511285096538));
#8320=CARTESIAN_POINT('Ctrl Pts',(0.548874290046456,-0.159766064500479,
0.813159949759));
#8321=CARTESIAN_POINT('Ctrl Pts',(0.573915184558107,-0.190326085855194,
0.795684265985089));
#8322=CARTESIAN_POINT('Ctrl Pts',(0.587792702767295,-0.203463743702801,
0.78555112003688));
#8323=CARTESIAN_POINT('Ctrl Pts',(0.615966552324775,-0.224161999508995,
0.763642258217233));
#8324=CARTESIAN_POINT('Ctrl Pts',(0.631684198665438,-0.232861760990032,
0.750785745543687));
#8325=CARTESIAN_POINT('Ctrl Pts',(0.663382628119203,-0.244251601209411,
0.722929908501543));
#8326=CARTESIAN_POINT('Ctrl Pts',(0.679352081686668,-0.246942143572133,
0.707917883896095));
#8327=CARTESIAN_POINT('Ctrl Pts',(0.707917883896095,-0.246942143572133,
0.679352081686668));
#8328=CARTESIAN_POINT('Ctrl Pts',(0.722929908501543,-0.244251601209411,
0.663382628119203));
#8329=CARTESIAN_POINT('Ctrl Pts',(0.750785745543687,-0.232861760990032,
0.631684198665439));
#8330=CARTESIAN_POINT('Ctrl Pts',(0.763642258217232,-0.224161999508995,
0.615966552324775));
#8331=CARTESIAN_POINT('Ctrl Pts',(0.78555112003688,-0.203463743702801,0.587792702767295));
#8332=CARTESIAN_POINT('Ctrl Pts',(0.795684265985088,-0.190326085855194,
0.573915184558108));
#8333=CARTESIAN_POINT('Ctrl Pts',(0.813159949759,-0.15976606450048,0.548874290046456));
#8334=CARTESIAN_POINT('Ctrl Pts',(0.820511285096538,-0.142345102874864,
0.537715343527944));
#8335=CARTESIAN_POINT('Ctrl Pts',(0.833661031856294,-0.099930567888331,
0.517157748491653));
#8336=CARTESIAN_POINT('Ctrl Pts',(0.838633903678357,-0.0740444353928835,
0.508899795931835));
#8337=CARTESIAN_POINT('Ctrl Pts',(0.841298510752801,-0.0476299999999999,
0.504455939115715));
#8338=CARTESIAN_POINT('',(0.528110872004958,-0.04763,0.871530771444223));
#8339=CARTESIAN_POINT('Origin',(0.707106781186547,-0.04763,0.707106781186548));
#8340=CARTESIAN_POINT('',(0.871530771444223,-0.04763,0.528110872004959));
#8341=CARTESIAN_POINT('Ctrl Pts',(0.871530771444223,-0.0476300000000001,
0.528110872004958));
#8342=CARTESIAN_POINT('Ctrl Pts',(0.87014664509073,-0.0609922781173483,
0.530395067942936));
#8343=CARTESIAN_POINT('Ctrl Pts',(0.868149331745851,-0.0742967091364493,
0.533674141594226));
#8344=CARTESIAN_POINT('Ctrl Pts',(0.85981294420286,-0.115492077056649,0.54708917182331));
#8345=CARTESIAN_POINT('Ctrl Pts',(0.850993704737257,-0.141695629206859,
0.560922177770136));
#8346=CARTESIAN_POINT('Ctrl Pts',(0.830754510485543,-0.181890537957859,
0.590422647829571));
#8347=CARTESIAN_POINT('Ctrl Pts',(0.816896541396381,-0.201072148666545,
0.609616703125488));
#8348=CARTESIAN_POINT('Ctrl Pts',(0.792310597819928,-0.223955109275652,
0.641117951819998));
#8349=CARTESIAN_POINT('Ctrl Pts',(0.779109323683612,-0.232742381310829,
0.657208095763053));
#8350=CARTESIAN_POINT('Ctrl Pts',(0.750552691816206,-0.244234834628584,
0.68964083160521));
#8351=CARTESIAN_POINT('Ctrl Pts',(0.735185187071673,-0.246942143572133,
0.705971972091755));
#8352=CARTESIAN_POINT('Ctrl Pts',(0.705971972091754,-0.246942143572133,
0.735185187071673));
#8353=CARTESIAN_POINT('Ctrl Pts',(0.689640831605209,-0.244234834628584,
0.750552691816206));
#8354=CARTESIAN_POINT('Ctrl Pts',(0.657208095763052,-0.232742381310829,
0.779109323683612));
#8355=CARTESIAN_POINT('Ctrl Pts',(0.641117951819998,-0.223955109275652,
0.792310597819928));
#8356=CARTESIAN_POINT('Ctrl Pts',(0.609616703125487,-0.201072148666545,
0.816896541396382));
#8357=CARTESIAN_POINT('Ctrl Pts',(0.590422647829571,-0.181890537957858,
0.830754510485544));
#8358=CARTESIAN_POINT('Ctrl Pts',(0.560922177770135,-0.141695629206858,
0.850993704737257));
#8359=CARTESIAN_POINT('Ctrl Pts',(0.547089171823309,-0.115492077056649,
0.859812944202861));
#8360=CARTESIAN_POINT('Ctrl Pts',(0.533674141594226,-0.0742967091364491,
0.868149331745852));
#8361=CARTESIAN_POINT('Ctrl Pts',(0.530395067942936,-0.0609922781173483,
0.870146645090731));
#8362=CARTESIAN_POINT('Ctrl Pts',(0.528110872004958,-0.0476300000000001,
0.871530771444223));
#8363=CARTESIAN_POINT('Origin',(0.707106781186547,-0.04763,0.707106781186548));
#8364=CARTESIAN_POINT('Origin',(0.,-0.166705,0.));
#8365=CARTESIAN_POINT('',(0.242834539687906,-0.04763,0.989696097314));
#8366=CARTESIAN_POINT('Origin',(0.,-0.04763,0.));
#8367=CARTESIAN_POINT('',(-0.242834539687907,-0.04763,0.989696097314));
#8368=CARTESIAN_POINT('Ctrl Pts',(0.242834539687906,-0.04763,0.989696097314));
#8369=CARTESIAN_POINT('Ctrl Pts',(0.24024064412003,-0.0609922781173483,
0.990332542620729));
#8370=CARTESIAN_POINT('Ctrl Pts',(0.236509675094874,-0.0742967091364492,
0.991238884025248));
#8371=CARTESIAN_POINT('Ctrl Pts',(0.221129100087819,-0.115492077056649,
0.994830026707808));
#8372=CARTESIAN_POINT('Ctrl Pts',(0.205111543747588,-0.141695629206859,
0.998375294985966));
#8373=CARTESIAN_POINT('Ctrl Pts',(0.169940289819232,-0.181890537957859,
1.00492400591205));
#8374=CARTESIAN_POINT('Ctrl Pts',(0.1465689792446,-0.201072148666545,1.00869718865384));
#8375=CARTESIAN_POINT('Ctrl Pts',(0.106909345252087,-0.223955109275652,
1.01358704779679));
#8376=CARTESIAN_POINT('Ctrl Pts',(0.0861971848975941,-0.232742381310829,
1.0156297872271));
#8377=CARTESIAN_POINT('Ctrl Pts',(0.0430711894098822,-0.244234834628584,
1.01837060663223));
#8378=CARTESIAN_POINT('Ctrl Pts',(0.0206568624125605,-0.246942143572133,
1.019052));
#8379=CARTESIAN_POINT('Ctrl Pts',(-0.0206568624125608,-0.246942143572133,
1.019052));
#8380=CARTESIAN_POINT('Ctrl Pts',(-0.0430711894098825,-0.244234834628584,
1.01837060663223));
#8381=CARTESIAN_POINT('Ctrl Pts',(-0.0861971848975943,-0.232742381310829,
1.0156297872271));
#8382=CARTESIAN_POINT('Ctrl Pts',(-0.106909345252088,-0.223955109275652,
1.01358704779679));
#8383=CARTESIAN_POINT('Ctrl Pts',(-0.1465689792446,-0.201072148666545,1.00869718865384));
#8384=CARTESIAN_POINT('Ctrl Pts',(-0.169940289819232,-0.181890537957859,
1.00492400591205));
#8385=CARTESIAN_POINT('Ctrl Pts',(-0.205111543747588,-0.141695629206859,
0.998375294985966));
#8386=CARTESIAN_POINT('Ctrl Pts',(-0.221129100087819,-0.115492077056649,
0.994830026707808));
#8387=CARTESIAN_POINT('Ctrl Pts',(-0.236509675094875,-0.0742967091364493,
0.991238884025248));
#8388=CARTESIAN_POINT('Ctrl Pts',(-0.24024064412003,-0.0609922781173483,
0.990332542620729));
#8389=CARTESIAN_POINT('Ctrl Pts',(-0.242834539687907,-0.04763,0.989696097314));
#8390=CARTESIAN_POINT('',(-0.528110872004959,-0.04763,0.871530771444223));
#8391=CARTESIAN_POINT('Origin',(0.,-0.04763,0.));
#8392=CARTESIAN_POINT('',(-0.871530771444223,-0.04763,0.528110872004958));
#8393=CARTESIAN_POINT('Ctrl Pts',(-0.528110872004958,-0.0476300000000001,
0.871530771444223));
#8394=CARTESIAN_POINT('Ctrl Pts',(-0.530395067942936,-0.0609922781173484,
0.87014664509073));
#8395=CARTESIAN_POINT('Ctrl Pts',(-0.533674141594226,-0.0742967091364493,
0.868149331745851));
#8396=CARTESIAN_POINT('Ctrl Pts',(-0.54708917182331,-0.115492077056649,
0.85981294420286));
#8397=CARTESIAN_POINT('Ctrl Pts',(-0.560922177770136,-0.141695629206859,
0.850993704737257));
#8398=CARTESIAN_POINT('Ctrl Pts',(-0.590422647829571,-0.181890537957859,
0.830754510485543));
#8399=CARTESIAN_POINT('Ctrl Pts',(-0.609616703125488,-0.201072148666545,
0.816896541396381));
#8400=CARTESIAN_POINT('Ctrl Pts',(-0.641117951819998,-0.223955109275652,
0.792310597819928));
#8401=CARTESIAN_POINT('Ctrl Pts',(-0.657208095763053,-0.232742381310829,
0.779109323683611));
#8402=CARTESIAN_POINT('Ctrl Pts',(-0.68964083160521,-0.244234834628584,
0.750552691816205));
#8403=CARTESIAN_POINT('Ctrl Pts',(-0.705971972091755,-0.246942143572133,
0.735185187071673));
#8404=CARTESIAN_POINT('Ctrl Pts',(-0.735185187071673,-0.246942143572133,
0.705971972091754));
#8405=CARTESIAN_POINT('Ctrl Pts',(-0.750552691816206,-0.244234834628584,
0.689640831605209));
#8406=CARTESIAN_POINT('Ctrl Pts',(-0.779109323683612,-0.232742381310829,
0.657208095763052));
#8407=CARTESIAN_POINT('Ctrl Pts',(-0.792310597819928,-0.223955109275652,
0.641117951819998));
#8408=CARTESIAN_POINT('Ctrl Pts',(-0.816896541396382,-0.201072148666545,
0.609616703125487));
#8409=CARTESIAN_POINT('Ctrl Pts',(-0.830754510485544,-0.181890537957858,
0.590422647829571));
#8410=CARTESIAN_POINT('Ctrl Pts',(-0.850993704737257,-0.141695629206858,
0.560922177770135));
#8411=CARTESIAN_POINT('Ctrl Pts',(-0.859812944202861,-0.115492077056649,
0.547089171823309));
#8412=CARTESIAN_POINT('Ctrl Pts',(-0.868149331745852,-0.0742967091364491,
0.533674141594226));
#8413=CARTESIAN_POINT('Ctrl Pts',(-0.870146645090731,-0.0609922781173483,
0.530395067942936));
#8414=CARTESIAN_POINT('Ctrl Pts',(-0.871530771444223,-0.04763,0.528110872004958));
#8415=CARTESIAN_POINT('',(-0.989696097314,-0.04763,0.242834539687906));
#8416=CARTESIAN_POINT('Origin',(0.,-0.04763,0.));
#8417=CARTESIAN_POINT('',(-1.019052,-0.246942143572133,1.248489836334E-16));
#8418=CARTESIAN_POINT('Ctrl Pts',(-0.989696097314,-0.04763,0.242834539687906));
#8419=CARTESIAN_POINT('Ctrl Pts',(-0.990332542620729,-0.0609922781173483,
0.24024064412003));
#8420=CARTESIAN_POINT('Ctrl Pts',(-0.991238884025248,-0.0742967091364492,
0.236509675094874));
#8421=CARTESIAN_POINT('Ctrl Pts',(-0.994830026707808,-0.115492077056649,
0.221129100087819));
#8422=CARTESIAN_POINT('Ctrl Pts',(-0.998375294985966,-0.141695629206859,
0.205111543747588));
#8423=CARTESIAN_POINT('Ctrl Pts',(-1.00492400591205,-0.181890537957859,
0.169940289819232));
#8424=CARTESIAN_POINT('Ctrl Pts',(-1.00869718865384,-0.201072148666545,
0.1465689792446));
#8425=CARTESIAN_POINT('Ctrl Pts',(-1.01358704779679,-0.223955109275652,
0.106909345252088));
#8426=CARTESIAN_POINT('Ctrl Pts',(-1.0156297872271,-0.232742381310829,0.0861971848975944));
#8427=CARTESIAN_POINT('Ctrl Pts',(-1.01837060663223,-0.244234834628584,
0.0430711894098825));
#8428=CARTESIAN_POINT('Ctrl Pts',(-1.019052,-0.246942143572133,0.0206568624125608));
#8429=CARTESIAN_POINT('Ctrl Pts',(-1.019052,-0.246942143572133,1.2490009027033E-16));
#8430=CARTESIAN_POINT('',(-1.019052,-0.28578,1.24797876996471E-16));
#8431=CARTESIAN_POINT('',(-1.019052,-0.166705,1.24797876996471E-16));
#8432=CARTESIAN_POINT('Origin',(0.,-0.28578,0.));
#8433=CARTESIAN_POINT('',(-0.989696097314,-0.04763,-0.242834539687906));
#8434=CARTESIAN_POINT('Ctrl Pts',(-1.019052,-0.246942143572133,1.2490009027033E-16));
#8435=CARTESIAN_POINT('Ctrl Pts',(-1.019052,-0.246942143572133,-0.0206568624125605));
#8436=CARTESIAN_POINT('Ctrl Pts',(-1.01837060663223,-0.244234834628584,
-0.0430711894098822));
#8437=CARTESIAN_POINT('Ctrl Pts',(-1.0156297872271,-0.232742381310829,-0.0861971848975941));
#8438=CARTESIAN_POINT('Ctrl Pts',(-1.01358704779679,-0.223955109275652,
-0.106909345252087));
#8439=CARTESIAN_POINT('Ctrl Pts',(-1.00869718865384,-0.201072148666546,
-0.1465689792446));
#8440=CARTESIAN_POINT('Ctrl Pts',(-1.00492400591205,-0.181890537957859,
-0.169940289819232));
#8441=CARTESIAN_POINT('Ctrl Pts',(-0.998375294985966,-0.141695629206859,
-0.205111543747588));
#8442=CARTESIAN_POINT('Ctrl Pts',(-0.994830026707808,-0.11549207705665,
-0.221129100087819));
#8443=CARTESIAN_POINT('Ctrl Pts',(-0.991238884025248,-0.0742967091364495,
-0.236509675094874));
#8444=CARTESIAN_POINT('Ctrl Pts',(-0.990332542620729,-0.0609922781173484,
-0.24024064412003));
#8445=CARTESIAN_POINT('Ctrl Pts',(-0.989696097314,-0.0476300000000001,-0.242834539687907));
#8446=CARTESIAN_POINT('',(-0.871530771444223,-0.04763,-0.528110872004958));
#8447=CARTESIAN_POINT('Origin',(0.,-0.04763,0.));
#8448=CARTESIAN_POINT('',(-0.528110872004958,-0.04763,-0.871530771444223));
#8449=CARTESIAN_POINT('Ctrl Pts',(-0.871530771444223,-0.0476300000000001,
-0.528110872004958));
#8450=CARTESIAN_POINT('Ctrl Pts',(-0.87014664509073,-0.0609922781173484,
-0.530395067942936));
#8451=CARTESIAN_POINT('Ctrl Pts',(-0.868149331745851,-0.0742967091364494,
-0.533674141594226));
#8452=CARTESIAN_POINT('Ctrl Pts',(-0.85981294420286,-0.115492077056649,
-0.54708917182331));
#8453=CARTESIAN_POINT('Ctrl Pts',(-0.850993704737257,-0.141695629206859,
-0.560922177770136));
#8454=CARTESIAN_POINT('Ctrl Pts',(-0.830754510485543,-0.181890537957859,
-0.590422647829571));
#8455=CARTESIAN_POINT('Ctrl Pts',(-0.816896541396381,-0.201072148666546,
-0.609616703125488));
#8456=CARTESIAN_POINT('Ctrl Pts',(-0.792310597819928,-0.223955109275652,
-0.641117951819999));
#8457=CARTESIAN_POINT('Ctrl Pts',(-0.779109323683611,-0.232742381310829,
-0.657208095763053));
#8458=CARTESIAN_POINT('Ctrl Pts',(-0.750552691816205,-0.244234834628584,
-0.68964083160521));
#8459=CARTESIAN_POINT('Ctrl Pts',(-0.735185187071673,-0.246942143572133,
-0.705971972091755));
#8460=CARTESIAN_POINT('Ctrl Pts',(-0.705971972091754,-0.246942143572133,
-0.735185187071673));
#8461=CARTESIAN_POINT('Ctrl Pts',(-0.68964083160521,-0.244234834628584,
-0.750552691816206));
#8462=CARTESIAN_POINT('Ctrl Pts',(-0.657208095763052,-0.232742381310829,
-0.779109323683612));
#8463=CARTESIAN_POINT('Ctrl Pts',(-0.641117951819998,-0.223955109275652,
-0.792310597819928));
#8464=CARTESIAN_POINT('Ctrl Pts',(-0.609616703125488,-0.201072148666545,
-0.816896541396381));
#8465=CARTESIAN_POINT('Ctrl Pts',(-0.590422647829571,-0.181890537957859,
-0.830754510485543));
#8466=CARTESIAN_POINT('Ctrl Pts',(-0.560922177770136,-0.141695629206859,
-0.850993704737257));
#8467=CARTESIAN_POINT('Ctrl Pts',(-0.54708917182331,-0.115492077056649,
-0.85981294420286));
#8468=CARTESIAN_POINT('Ctrl Pts',(-0.533674141594226,-0.0742967091364494,
-0.868149331745852));
#8469=CARTESIAN_POINT('Ctrl Pts',(-0.530395067942936,-0.0609922781173484,
-0.870146645090731));
#8470=CARTESIAN_POINT('Ctrl Pts',(-0.528110872004958,-0.0476300000000001,
-0.871530771444223));
#8471=CARTESIAN_POINT('',(-0.242834539687906,-0.04763,-0.989696097314));
#8472=CARTESIAN_POINT('Origin',(0.,-0.04763,0.));
#8473=CARTESIAN_POINT('',(0.242834539687906,-0.04763,-0.989696097314));
#8474=CARTESIAN_POINT('Ctrl Pts',(-0.242834539687907,-0.04763,-0.989696097314));
#8475=CARTESIAN_POINT('Ctrl Pts',(-0.24024064412003,-0.0609922781173483,
-0.990332542620729));
#8476=CARTESIAN_POINT('Ctrl Pts',(-0.236509675094874,-0.0742967091364493,
-0.991238884025248));
#8477=CARTESIAN_POINT('Ctrl Pts',(-0.221129100087819,-0.115492077056649,
-0.994830026707808));
#8478=CARTESIAN_POINT('Ctrl Pts',(-0.205111543747588,-0.141695629206859,
-0.998375294985966));
#8479=CARTESIAN_POINT('Ctrl Pts',(-0.169940289819232,-0.181890537957859,
-1.00492400591205));
#8480=CARTESIAN_POINT('Ctrl Pts',(-0.1465689792446,-0.201072148666545,-1.00869718865384));
#8481=CARTESIAN_POINT('Ctrl Pts',(-0.106909345252087,-0.223955109275652,
-1.01358704779679));
#8482=CARTESIAN_POINT('Ctrl Pts',(-0.0861971848975942,-0.232742381310829,
-1.0156297872271));
#8483=CARTESIAN_POINT('Ctrl Pts',(-0.0430711894098823,-0.244234834628584,
-1.01837060663223));
#8484=CARTESIAN_POINT('Ctrl Pts',(-0.0206568624125606,-0.246942143572133,
-1.019052));
#8485=CARTESIAN_POINT('Ctrl Pts',(0.0206568624125607,-0.246942143572133,
-1.019052));
#8486=CARTESIAN_POINT('Ctrl Pts',(0.0430711894098824,-0.244234834628584,
-1.01837060663223));
#8487=CARTESIAN_POINT('Ctrl Pts',(0.0861971848975943,-0.232742381310829,
-1.0156297872271));
#8488=CARTESIAN_POINT('Ctrl Pts',(0.106909345252088,-0.223955109275652,
-1.01358704779679));
#8489=CARTESIAN_POINT('Ctrl Pts',(0.1465689792446,-0.201072148666545,-1.00869718865384));
#8490=CARTESIAN_POINT('Ctrl Pts',(0.169940289819232,-0.181890537957859,
-1.00492400591205));
#8491=CARTESIAN_POINT('Ctrl Pts',(0.205111543747588,-0.141695629206859,
-0.998375294985966));
#8492=CARTESIAN_POINT('Ctrl Pts',(0.221129100087819,-0.115492077056649,
-0.994830026707808));
#8493=CARTESIAN_POINT('Ctrl Pts',(0.236509675094874,-0.0742967091364493,
-0.991238884025248));
#8494=CARTESIAN_POINT('Ctrl Pts',(0.24024064412003,-0.0609922781173484,
-0.990332542620729));
#8495=CARTESIAN_POINT('Ctrl Pts',(0.242834539687907,-0.04763,-0.989696097314));
#8496=CARTESIAN_POINT('',(0.528110872004958,-0.04763,-0.871530771444223));
#8497=CARTESIAN_POINT('Origin',(0.,-0.04763,0.));
#8498=CARTESIAN_POINT('',(0.871530771444223,-0.04763,-0.528110872004958));
#8499=CARTESIAN_POINT('Ctrl Pts',(0.528110872004958,-0.0476300000000001,
-0.871530771444223));
#8500=CARTESIAN_POINT('Ctrl Pts',(0.530395067942936,-0.0609922781173484,
-0.870146645090731));
#8501=CARTESIAN_POINT('Ctrl Pts',(0.533674141594226,-0.0742967091364493,
-0.868149331745851));
#8502=CARTESIAN_POINT('Ctrl Pts',(0.54708917182331,-0.115492077056649,-0.85981294420286));
#8503=CARTESIAN_POINT('Ctrl Pts',(0.560922177770136,-0.141695629206859,
-0.850993704737257));
#8504=CARTESIAN_POINT('Ctrl Pts',(0.590422647829571,-0.181890537957859,
-0.830754510485543));
#8505=CARTESIAN_POINT('Ctrl Pts',(0.609616703125488,-0.201072148666545,
-0.816896541396381));
#8506=CARTESIAN_POINT('Ctrl Pts',(0.641117951819998,-0.223955109275652,
-0.792310597819928));
#8507=CARTESIAN_POINT('Ctrl Pts',(0.657208095763053,-0.232742381310829,
-0.779109323683612));
#8508=CARTESIAN_POINT('Ctrl Pts',(0.68964083160521,-0.244234834628584,-0.750552691816206));
#8509=CARTESIAN_POINT('Ctrl Pts',(0.705971972091755,-0.246942143572133,
-0.735185187071673));
#8510=CARTESIAN_POINT('Ctrl Pts',(0.735185187071673,-0.246942143572133,
-0.705971972091754));
#8511=CARTESIAN_POINT('Ctrl Pts',(0.750552691816206,-0.244234834628584,
-0.68964083160521));
#8512=CARTESIAN_POINT('Ctrl Pts',(0.779109323683612,-0.232742381310829,
-0.657208095763053));
#8513=CARTESIAN_POINT('Ctrl Pts',(0.792310597819928,-0.223955109275652,
-0.641117951819998));
#8514=CARTESIAN_POINT('Ctrl Pts',(0.816896541396381,-0.201072148666545,
-0.609616703125488));
#8515=CARTESIAN_POINT('Ctrl Pts',(0.830754510485543,-0.181890537957859,
-0.590422647829571));
#8516=CARTESIAN_POINT('Ctrl Pts',(0.850993704737257,-0.141695629206859,
-0.560922177770136));
#8517=CARTESIAN_POINT('Ctrl Pts',(0.85981294420286,-0.115492077056649,-0.54708917182331));
#8518=CARTESIAN_POINT('Ctrl Pts',(0.868149331745851,-0.0742967091364493,
-0.533674141594226));
#8519=CARTESIAN_POINT('Ctrl Pts',(0.870146645090731,-0.0609922781173484,
-0.530395067942936));
#8520=CARTESIAN_POINT('Ctrl Pts',(0.871530771444223,-0.0476300000000001,
-0.528110872004958));
#8521=CARTESIAN_POINT('',(0.989696097314,-0.04763,-0.242834539687906));
#8522=CARTESIAN_POINT('Origin',(0.,-0.04763,0.));
#8523=CARTESIAN_POINT('',(0.989696097314,-0.04763,0.242834539687906));
#8524=CARTESIAN_POINT('Ctrl Pts',(0.989696097314,-0.04763,-0.242834539687907));
#8525=CARTESIAN_POINT('Ctrl Pts',(0.990332542620729,-0.0609922781173483,
-0.24024064412003));
#8526=CARTESIAN_POINT('Ctrl Pts',(0.991238884025248,-0.0742967091364493,
-0.236509675094874));
#8527=CARTESIAN_POINT('Ctrl Pts',(0.994830026707808,-0.115492077056649,
-0.221129100087819));
#8528=CARTESIAN_POINT('Ctrl Pts',(0.998375294985966,-0.141695629206859,
-0.205111543747588));
#8529=CARTESIAN_POINT('Ctrl Pts',(1.00492400591205,-0.181890537957859,-0.169940289819232));
#8530=CARTESIAN_POINT('Ctrl Pts',(1.00869718865384,-0.201072148666545,-0.1465689792446));
#8531=CARTESIAN_POINT('Ctrl Pts',(1.01358704779679,-0.223955109275652,-0.106909345252087));
#8532=CARTESIAN_POINT('Ctrl Pts',(1.0156297872271,-0.232742381310829,-0.0861971848975942));
#8533=CARTESIAN_POINT('Ctrl Pts',(1.01837060663223,-0.244234834628584,-0.0430711894098823));
#8534=CARTESIAN_POINT('Ctrl Pts',(1.019052,-0.246942143572133,-0.0206568624125607));
#8535=CARTESIAN_POINT('Ctrl Pts',(1.019052,-0.246942143572133,0.0206568624125607));
#8536=CARTESIAN_POINT('Ctrl Pts',(1.01837060663223,-0.244234834628584,0.0430711894098823));
#8537=CARTESIAN_POINT('Ctrl Pts',(1.0156297872271,-0.232742381310829,0.0861971848975942));
#8538=CARTESIAN_POINT('Ctrl Pts',(1.01358704779679,-0.223955109275652,0.106909345252087));
#8539=CARTESIAN_POINT('Ctrl Pts',(1.00869718865384,-0.201072148666545,0.1465689792446));
#8540=CARTESIAN_POINT('Ctrl Pts',(1.00492400591205,-0.181890537957859,0.169940289819232));
#8541=CARTESIAN_POINT('Ctrl Pts',(0.998375294985966,-0.141695629206859,
0.205111543747588));
#8542=CARTESIAN_POINT('Ctrl Pts',(0.994830026707808,-0.115492077056649,
0.221129100087819));
#8543=CARTESIAN_POINT('Ctrl Pts',(0.991238884025248,-0.0742967091364492,
0.236509675094874));
#8544=CARTESIAN_POINT('Ctrl Pts',(0.990332542620729,-0.0609922781173483,
0.24024064412003));
#8545=CARTESIAN_POINT('Ctrl Pts',(0.989696097314,-0.04763,0.242834539687907));
#8546=CARTESIAN_POINT('Origin',(0.,-0.04763,0.));
#8547=CARTESIAN_POINT('Origin',(0.,-0.04763,0.));
#8548=CARTESIAN_POINT('',(0.238183666596899,-0.04763,0.951592097314));
#8549=CARTESIAN_POINT('Origin',(0.,-0.04763,0.));
#8550=CARTESIAN_POINT('Origin',(-1.94289029309402E-16,-0.04763,1.));
#8551=CARTESIAN_POINT('Origin',(-1.94289029309402E-16,0.,1.));
#8552=CARTESIAN_POINT('',(-0.2381836665969,-0.04763,0.951592097314));
#8553=CARTESIAN_POINT('Ctrl Pts',(-0.238183666596899,-0.0476299999999999,
0.951592097314));
#8554=CARTESIAN_POINT('Ctrl Pts',(-0.233157223576062,-0.0740444353928835,
0.952850216871763));
#8555=CARTESIAN_POINT('Ctrl Pts',(-0.223801617934946,-0.0999305678883309,
0.955173119738174));
#8556=CARTESIAN_POINT('Ctrl Pts',(-0.199966927975188,-0.142345102874864,
0.960411259488514));
#8557=CARTESIAN_POINT('Ctrl Pts',(-0.1868781821531,-0.159766064500479,0.963103647174702));
#8558=CARTESIAN_POINT('Ctrl Pts',(-0.15681442133453,-0.190326085855194,
0.968453058988463));
#8559=CARTESIAN_POINT('Ctrl Pts',(-0.139836317888043,-0.203463743702801,
0.971100730005489));
#8560=CARTESIAN_POINT('Ctrl Pts',(-0.104422493053067,-0.224161999508995,
0.975530745318961));
#8561=CARTESIAN_POINT('Ctrl Pts',(-0.0842175114474176,-0.232861760990032,
0.977553872336861));
#8562=CARTESIAN_POINT('Ctrl Pts',(-0.0421062857595701,-0.244251601209411,
0.980270995488453));
#8563=CARTESIAN_POINT('Ctrl Pts',(-0.0201990724523197,-0.246942143572133,
0.980948));
#8564=CARTESIAN_POINT('Ctrl Pts',(0.020199072452319,-0.246942143572133,
0.980948));
#8565=CARTESIAN_POINT('Ctrl Pts',(0.0421062857595694,-0.244251601209411,
0.980270995488454));
#8566=CARTESIAN_POINT('Ctrl Pts',(0.0842175114474169,-0.232861760990032,
0.977553872336861));
#8567=CARTESIAN_POINT('Ctrl Pts',(0.104422493053067,-0.224161999508995,
0.975530745318961));
#8568=CARTESIAN_POINT('Ctrl Pts',(0.139836317888042,-0.203463743702801,
0.971100730005489));
#8569=CARTESIAN_POINT('Ctrl Pts',(0.15681442133453,-0.190326085855194,0.968453058988463));
#8570=CARTESIAN_POINT('Ctrl Pts',(0.1868781821531,-0.15976606450048,0.963103647174702));
#8571=CARTESIAN_POINT('Ctrl Pts',(0.199966927975188,-0.142345102874864,
0.960411259488514));
#8572=CARTESIAN_POINT('Ctrl Pts',(0.223801617934945,-0.0999305678883309,
0.955173119738174));
#8573=CARTESIAN_POINT('Ctrl Pts',(0.233157223576061,-0.0740444353928835,
0.952850216871763));
#8574=CARTESIAN_POINT('Ctrl Pts',(0.238183666596899,-0.0476299999999999,
0.951592097314));
#8575=CARTESIAN_POINT('Origin',(-1.94289029309402E-16,-0.04763,1.));
#8576=CARTESIAN_POINT('Origin',(0.,-0.04763,0.));
#8577=CARTESIAN_POINT('',(-0.504455939115715,-0.04763,0.841298510752802));
#8578=CARTESIAN_POINT('Origin',(0.,-0.04763,0.));
#8579=CARTESIAN_POINT('Origin',(-0.707106781186548,-0.04763,0.707106781186547));
#8580=CARTESIAN_POINT('Origin',(-0.707106781186548,0.,0.707106781186547));
#8581=CARTESIAN_POINT('',(-0.841298510752802,-0.04763,0.504455939115715));
#8582=CARTESIAN_POINT('Ctrl Pts',(-0.841298510752802,-0.04763,0.504455939115715));
#8583=CARTESIAN_POINT('Ctrl Pts',(-0.838633903678357,-0.0740444353928835,
0.508899795931835));
#8584=CARTESIAN_POINT('Ctrl Pts',(-0.833661031856294,-0.0999305678883309,
0.517157748491652));
#8585=CARTESIAN_POINT('Ctrl Pts',(-0.820511285096538,-0.142345102874864,
0.537715343527944));
#8586=CARTESIAN_POINT('Ctrl Pts',(-0.813159949759,-0.159766064500479,0.548874290046456));
#8587=CARTESIAN_POINT('Ctrl Pts',(-0.795684265985089,-0.190326085855194,
0.573915184558107));
#8588=CARTESIAN_POINT('Ctrl Pts',(-0.78555112003688,-0.203463743702801,
0.587792702767295));
#8589=CARTESIAN_POINT('Ctrl Pts',(-0.763642258217233,-0.224161999508995,
0.615966552324775));
#8590=CARTESIAN_POINT('Ctrl Pts',(-0.750785745543687,-0.232861760990032,
0.631684198665438));
#8591=CARTESIAN_POINT('Ctrl Pts',(-0.722929908501543,-0.244251601209411,
0.663382628119203));
#8592=CARTESIAN_POINT('Ctrl Pts',(-0.707917883896095,-0.246942143572133,
0.679352081686668));
#8593=CARTESIAN_POINT('Ctrl Pts',(-0.679352081686668,-0.246942143572133,
0.707917883896095));
#8594=CARTESIAN_POINT('Ctrl Pts',(-0.663382628119203,-0.244251601209411,
0.722929908501544));
#8595=CARTESIAN_POINT('Ctrl Pts',(-0.631684198665438,-0.232861760990031,
0.750785745543687));
#8596=CARTESIAN_POINT('Ctrl Pts',(-0.615966552324775,-0.224161999508995,
0.763642258217233));
#8597=CARTESIAN_POINT('Ctrl Pts',(-0.587792702767295,-0.203463743702801,
0.78555112003688));
#8598=CARTESIAN_POINT('Ctrl Pts',(-0.573915184558107,-0.190326085855194,
0.795684265985088));
#8599=CARTESIAN_POINT('Ctrl Pts',(-0.548874290046456,-0.159766064500479,
0.813159949759));
#8600=CARTESIAN_POINT('Ctrl Pts',(-0.537715343527944,-0.142345102874864,
0.820511285096538));
#8601=CARTESIAN_POINT('Ctrl Pts',(-0.517157748491652,-0.0999305678883309,
0.833661031856294));
#8602=CARTESIAN_POINT('Ctrl Pts',(-0.508899795931835,-0.0740444353928835,
0.838633903678357));
#8603=CARTESIAN_POINT('Ctrl Pts',(-0.504455939115716,-0.04763,0.841298510752801));
#8604=CARTESIAN_POINT('Origin',(-0.707106781186548,-0.04763,0.707106781186547));
#8605=CARTESIAN_POINT('Origin',(0.,-0.04763,0.));
#8606=CARTESIAN_POINT('',(-0.951592097314,-0.04763,0.238183666596899));
#8607=CARTESIAN_POINT('Origin',(0.,-0.04763,0.));
#8608=CARTESIAN_POINT('Origin',(-1.,-0.04763,-1.11022302462516E-16));
#8609=CARTESIAN_POINT('Origin',(-1.,0.,-1.11022302462516E-16));
#8610=CARTESIAN_POINT('',(-0.951592097314,-0.04763,-0.2381836665969));
#8611=CARTESIAN_POINT('',(-0.980948,-0.246942143572133,1.08514323328844E-18));
#8612=CARTESIAN_POINT('Ctrl Pts',(-0.951592097314,-0.04763,-0.238183666596899));
#8613=CARTESIAN_POINT('Ctrl Pts',(-0.952850216871763,-0.0740444353928835,
-0.233157223576062));
#8614=CARTESIAN_POINT('Ctrl Pts',(-0.955173119738174,-0.0999305678883309,
-0.223801617934946));
#8615=CARTESIAN_POINT('Ctrl Pts',(-0.960411259488514,-0.142345102874864,
-0.199966927975188));
#8616=CARTESIAN_POINT('Ctrl Pts',(-0.963103647174702,-0.159766064500479,
-0.1868781821531));
#8617=CARTESIAN_POINT('Ctrl Pts',(-0.968453058988463,-0.190326085855194,
-0.15681442133453));
#8618=CARTESIAN_POINT('Ctrl Pts',(-0.971100730005489,-0.203463743702801,
-0.139836317888043));
#8619=CARTESIAN_POINT('Ctrl Pts',(-0.975530745318961,-0.224161999508995,
-0.104422493053067));
#8620=CARTESIAN_POINT('Ctrl Pts',(-0.977553872336861,-0.232861760990032,
-0.0842175114474175));
#8621=CARTESIAN_POINT('Ctrl Pts',(-0.980270995488453,-0.244251601209411,
-0.0421062857595699));
#8622=CARTESIAN_POINT('Ctrl Pts',(-0.980948,-0.246942143572133,-0.0201990724523195));
#8623=CARTESIAN_POINT('Ctrl Pts',(-0.980948,-0.246942143572133,-1.17961196366423E-16));
#8624=CARTESIAN_POINT('Origin',(-1.,-0.04763,-1.11022302462516E-16));
#8625=CARTESIAN_POINT('Ctrl Pts',(-0.980948,-0.246942143572133,-1.17961196366423E-16));
#8626=CARTESIAN_POINT('Ctrl Pts',(-0.980948,-0.246942143572133,0.0201990724523192));
#8627=CARTESIAN_POINT('Ctrl Pts',(-0.980270995488453,-0.244251601209411,
0.0421062857595695));
#8628=CARTESIAN_POINT('Ctrl Pts',(-0.977553872336861,-0.232861760990032,
0.0842175114474169));
#8629=CARTESIAN_POINT('Ctrl Pts',(-0.975530745318961,-0.224161999508995,
0.104422493053066));
#8630=CARTESIAN_POINT('Ctrl Pts',(-0.971100730005489,-0.203463743702801,
0.139836317888042));
#8631=CARTESIAN_POINT('Ctrl Pts',(-0.968453058988463,-0.190326085855194,
0.15681442133453));
#8632=CARTESIAN_POINT('Ctrl Pts',(-0.963103647174702,-0.15976606450048,
0.1868781821531));
#8633=CARTESIAN_POINT('Ctrl Pts',(-0.960411259488514,-0.142345102874864,
0.199966927975188));
#8634=CARTESIAN_POINT('Ctrl Pts',(-0.955173119738174,-0.099930567888331,
0.223801617934945));
#8635=CARTESIAN_POINT('Ctrl Pts',(-0.952850216871763,-0.0740444353928835,
0.233157223576061));
#8636=CARTESIAN_POINT('Ctrl Pts',(-0.951592097314,-0.04763,0.238183666596899));
#8637=CARTESIAN_POINT('Origin',(0.,-0.04763,0.));
#8638=CARTESIAN_POINT('',(-0.841298510752802,-0.04763,-0.504455939115715));
#8639=CARTESIAN_POINT('Origin',(0.,-0.04763,0.));
#8640=CARTESIAN_POINT('Origin',(-0.707106781186547,-0.04763,-0.707106781186548));
#8641=CARTESIAN_POINT('Origin',(-0.707106781186547,0.,-0.707106781186548));
#8642=CARTESIAN_POINT('',(-0.504455939115715,-0.04763,-0.841298510752802));
#8643=CARTESIAN_POINT('Ctrl Pts',(-0.504455939115715,-0.04763,-0.841298510752802));
#8644=CARTESIAN_POINT('Ctrl Pts',(-0.508899795931835,-0.0740444353928835,
-0.838633903678357));
#8645=CARTESIAN_POINT('Ctrl Pts',(-0.517157748491652,-0.0999305678883309,
-0.833661031856294));
#8646=CARTESIAN_POINT('Ctrl Pts',(-0.537715343527944,-0.142345102874864,
-0.820511285096538));
#8647=CARTESIAN_POINT('Ctrl Pts',(-0.548874290046456,-0.159766064500479,
-0.813159949759));
#8648=CARTESIAN_POINT('Ctrl Pts',(-0.573915184558107,-0.190326085855194,
-0.795684265985089));
#8649=CARTESIAN_POINT('Ctrl Pts',(-0.587792702767295,-0.203463743702801,
-0.78555112003688));
#8650=CARTESIAN_POINT('Ctrl Pts',(-0.615966552324775,-0.224161999508995,
-0.763642258217233));
#8651=CARTESIAN_POINT('Ctrl Pts',(-0.631684198665438,-0.232861760990032,
-0.750785745543687));
#8652=CARTESIAN_POINT('Ctrl Pts',(-0.663382628119203,-0.244251601209411,
-0.722929908501543));
#8653=CARTESIAN_POINT('Ctrl Pts',(-0.679352081686668,-0.246942143572133,
-0.707917883896095));
#8654=CARTESIAN_POINT('Ctrl Pts',(-0.707917883896095,-0.246942143572133,
-0.679352081686668));
#8655=CARTESIAN_POINT('Ctrl Pts',(-0.722929908501543,-0.244251601209411,
-0.663382628119203));
#8656=CARTESIAN_POINT('Ctrl Pts',(-0.750785745543687,-0.232861760990032,
-0.631684198665439));
#8657=CARTESIAN_POINT('Ctrl Pts',(-0.763642258217232,-0.224161999508995,
-0.615966552324775));
#8658=CARTESIAN_POINT('Ctrl Pts',(-0.78555112003688,-0.203463743702801,
-0.587792702767295));
#8659=CARTESIAN_POINT('Ctrl Pts',(-0.795684265985088,-0.190326085855194,
-0.573915184558107));
#8660=CARTESIAN_POINT('Ctrl Pts',(-0.813159949759,-0.15976606450048,-0.548874290046456));
#8661=CARTESIAN_POINT('Ctrl Pts',(-0.820511285096538,-0.142345102874864,
-0.537715343527944));
#8662=CARTESIAN_POINT('Ctrl Pts',(-0.833661031856294,-0.0999305678883311,
-0.517157748491652));
#8663=CARTESIAN_POINT('Ctrl Pts',(-0.838633903678357,-0.0740444353928836,
-0.508899795931835));
#8664=CARTESIAN_POINT('Ctrl Pts',(-0.841298510752801,-0.04763,-0.504455939115715));
#8665=CARTESIAN_POINT('Origin',(-0.707106781186547,-0.04763,-0.707106781186548));
#8666=CARTESIAN_POINT('Origin',(0.,-0.04763,0.));
#8667=CARTESIAN_POINT('',(-0.238183666596899,-0.04763,-0.951592097314));
#8668=CARTESIAN_POINT('Origin',(0.,-0.04763,0.));
#8669=CARTESIAN_POINT('Origin',(5.55111512312578E-17,-0.04763,-1.));
#8670=CARTESIAN_POINT('Origin',(5.55111512312578E-17,0.,-1.));
#8671=CARTESIAN_POINT('',(0.238183666596899,-0.04763,-0.951592097314));
#8672=CARTESIAN_POINT('Ctrl Pts',(0.238183666596899,-0.04763,-0.951592097314));
#8673=CARTESIAN_POINT('Ctrl Pts',(0.233157223576062,-0.0740444353928835,
-0.952850216871763));
#8674=CARTESIAN_POINT('Ctrl Pts',(0.223801617934946,-0.099930567888331,
-0.955173119738174));
#8675=CARTESIAN_POINT('Ctrl Pts',(0.199966927975188,-0.142345102874864,
-0.960411259488514));
#8676=CARTESIAN_POINT('Ctrl Pts',(0.1868781821531,-0.15976606450048,-0.963103647174702));
#8677=CARTESIAN_POINT('Ctrl Pts',(0.15681442133453,-0.190326085855194,-0.968453058988463));
#8678=CARTESIAN_POINT('Ctrl Pts',(0.139836317888042,-0.203463743702801,
-0.971100730005489));
#8679=CARTESIAN_POINT('Ctrl Pts',(0.104422493053067,-0.224161999508995,
-0.975530745318961));
#8680=CARTESIAN_POINT('Ctrl Pts',(0.0842175114474173,-0.232861760990032,
-0.977553872336861));
#8681=CARTESIAN_POINT('Ctrl Pts',(0.0421062857595698,-0.244251601209411,
-0.980270995488453));
#8682=CARTESIAN_POINT('Ctrl Pts',(0.0201990724523194,-0.246942143572133,
-0.980948));
#8683=CARTESIAN_POINT('Ctrl Pts',(-0.0201990724523193,-0.246942143572133,
-0.980948));
#8684=CARTESIAN_POINT('Ctrl Pts',(-0.0421062857595697,-0.244251601209411,
-0.980270995488453));
#8685=CARTESIAN_POINT('Ctrl Pts',(-0.0842175114474171,-0.232861760990032,
-0.977553872336861));
#8686=CARTESIAN_POINT('Ctrl Pts',(-0.104422493053067,-0.224161999508995,
-0.975530745318961));
#8687=CARTESIAN_POINT('Ctrl Pts',(-0.139836317888042,-0.203463743702801,
-0.971100730005489));
#8688=CARTESIAN_POINT('Ctrl Pts',(-0.15681442133453,-0.190326085855194,
-0.968453058988463));
#8689=CARTESIAN_POINT('Ctrl Pts',(-0.1868781821531,-0.15976606450048,-0.963103647174702));
#8690=CARTESIAN_POINT('Ctrl Pts',(-0.199966927975188,-0.142345102874864,
-0.960411259488514));
#8691=CARTESIAN_POINT('Ctrl Pts',(-0.223801617934945,-0.099930567888331,
-0.955173119738174));
#8692=CARTESIAN_POINT('Ctrl Pts',(-0.233157223576062,-0.0740444353928835,
-0.952850216871763));
#8693=CARTESIAN_POINT('Ctrl Pts',(-0.238183666596899,-0.0476299999999999,
-0.951592097314));
#8694=CARTESIAN_POINT('Origin',(5.55111512312578E-17,-0.04763,-1.));
#8695=CARTESIAN_POINT('Origin',(0.,-0.04763,0.));
#8696=CARTESIAN_POINT('',(0.504455939115715,-0.04763,-0.841298510752802));
#8697=CARTESIAN_POINT('Origin',(0.,-0.04763,0.));
#8698=CARTESIAN_POINT('Origin',(0.707106781186548,-0.04763,-0.707106781186547));
#8699=CARTESIAN_POINT('Origin',(0.707106781186548,0.,-0.707106781186547));
#8700=CARTESIAN_POINT('',(0.841298510752802,-0.04763,-0.504455939115715));
#8701=CARTESIAN_POINT('Ctrl Pts',(0.841298510752802,-0.04763,-0.504455939115715));
#8702=CARTESIAN_POINT('Ctrl Pts',(0.838633903678357,-0.0740444353928835,
-0.508899795931835));
#8703=CARTESIAN_POINT('Ctrl Pts',(0.833661031856294,-0.0999305678883309,
-0.517157748491652));
#8704=CARTESIAN_POINT('Ctrl Pts',(0.820511285096538,-0.142345102874864,
-0.537715343527944));
#8705=CARTESIAN_POINT('Ctrl Pts',(0.813159949759,-0.159766064500479,-0.548874290046456));
#8706=CARTESIAN_POINT('Ctrl Pts',(0.795684265985088,-0.190326085855194,
-0.573915184558107));
#8707=CARTESIAN_POINT('Ctrl Pts',(0.78555112003688,-0.203463743702801,-0.587792702767295));
#8708=CARTESIAN_POINT('Ctrl Pts',(0.763642258217233,-0.224161999508995,
-0.615966552324775));
#8709=CARTESIAN_POINT('Ctrl Pts',(0.750785745543687,-0.232861760990032,
-0.631684198665438));
#8710=CARTESIAN_POINT('Ctrl Pts',(0.722929908501543,-0.244251601209411,
-0.663382628119203));
#8711=CARTESIAN_POINT('Ctrl Pts',(0.707917883896095,-0.246942143572133,
-0.679352081686668));
#8712=CARTESIAN_POINT('Ctrl Pts',(0.679352081686668,-0.246942143572133,
-0.707917883896095));
#8713=CARTESIAN_POINT('Ctrl Pts',(0.663382628119203,-0.244251601209411,
-0.722929908501543));
#8714=CARTESIAN_POINT('Ctrl Pts',(0.631684198665438,-0.232861760990032,
-0.750785745543687));
#8715=CARTESIAN_POINT('Ctrl Pts',(0.615966552324775,-0.224161999508995,
-0.763642258217232));
#8716=CARTESIAN_POINT('Ctrl Pts',(0.587792702767295,-0.203463743702801,
-0.78555112003688));
#8717=CARTESIAN_POINT('Ctrl Pts',(0.573915184558107,-0.190326085855194,
-0.795684265985088));
#8718=CARTESIAN_POINT('Ctrl Pts',(0.548874290046456,-0.159766064500479,
-0.813159949759));
#8719=CARTESIAN_POINT('Ctrl Pts',(0.537715343527944,-0.142345102874864,
-0.820511285096538));
#8720=CARTESIAN_POINT('Ctrl Pts',(0.517157748491652,-0.099930567888331,
-0.833661031856294));
#8721=CARTESIAN_POINT('Ctrl Pts',(0.508899795931835,-0.0740444353928835,
-0.838633903678357));
#8722=CARTESIAN_POINT('Ctrl Pts',(0.504455939115715,-0.04763,-0.841298510752801));
#8723=CARTESIAN_POINT('Origin',(0.707106781186548,-0.04763,-0.707106781186547));
#8724=CARTESIAN_POINT('Origin',(0.,-0.166705,0.));
#8725=CARTESIAN_POINT('',(-0.980948,-0.28578,1.20131482833E-16));
#8726=CARTESIAN_POINT('Origin',(0.,-0.28578,0.));
#8727=CARTESIAN_POINT('',(-0.980948,-0.166705,1.20131482833E-16));
#8728=CARTESIAN_POINT('',(0.951592097314,-0.04763,0.238183666596899));
#8729=CARTESIAN_POINT('Origin',(0.,-0.04763,0.));
#8730=CARTESIAN_POINT('',(0.951592097314,-0.04763,-0.238183666596899));
#8731=CARTESIAN_POINT('Ctrl Pts',(0.951592097314,-0.04763,0.238183666596899));
#8732=CARTESIAN_POINT('Ctrl Pts',(0.952850216871763,-0.0740444353928835,
0.233157223576062));
#8733=CARTESIAN_POINT('Ctrl Pts',(0.955173119738174,-0.099930567888331,
0.223801617934945));
#8734=CARTESIAN_POINT('Ctrl Pts',(0.960411259488514,-0.142345102874864,
0.199966927975188));
#8735=CARTESIAN_POINT('Ctrl Pts',(0.963103647174702,-0.15976606450048,0.1868781821531));
#8736=CARTESIAN_POINT('Ctrl Pts',(0.968453058988463,-0.190326085855194,
0.15681442133453));
#8737=CARTESIAN_POINT('Ctrl Pts',(0.971100730005489,-0.203463743702801,
0.139836317888042));
#8738=CARTESIAN_POINT('Ctrl Pts',(0.975530745318961,-0.224161999508995,
0.104422493053067));
#8739=CARTESIAN_POINT('Ctrl Pts',(0.977553872336861,-0.232861760990032,
0.0842175114474172));
#8740=CARTESIAN_POINT('Ctrl Pts',(0.980270995488453,-0.244251601209411,
0.0421062857595697));
#8741=CARTESIAN_POINT('Ctrl Pts',(0.980948,-0.246942143572133,0.0201990724523194));
#8742=CARTESIAN_POINT('Ctrl Pts',(0.980948,-0.246942143572133,-0.0201990724523194));
#8743=CARTESIAN_POINT('Ctrl Pts',(0.980270995488453,-0.244251601209411,
-0.0421062857595697));
#8744=CARTESIAN_POINT('Ctrl Pts',(0.977553872336861,-0.232861760990032,
-0.0842175114474172));
#8745=CARTESIAN_POINT('Ctrl Pts',(0.975530745318961,-0.224161999508995,
-0.104422493053067));
#8746=CARTESIAN_POINT('Ctrl Pts',(0.971100730005489,-0.203463743702801,
-0.139836317888042));
#8747=CARTESIAN_POINT('Ctrl Pts',(0.968453058988463,-0.190326085855194,
-0.15681442133453));
#8748=CARTESIAN_POINT('Ctrl Pts',(0.963103647174702,-0.15976606450048,-0.1868781821531));
#8749=CARTESIAN_POINT('Ctrl Pts',(0.960411259488514,-0.142345102874864,
-0.199966927975188));
#8750=CARTESIAN_POINT('Ctrl Pts',(0.955173119738174,-0.099930567888331,
-0.223801617934945));
#8751=CARTESIAN_POINT('Ctrl Pts',(0.952850216871763,-0.0740444353928835,
-0.233157223576062));
#8752=CARTESIAN_POINT('Ctrl Pts',(0.951592097314,-0.0476299999999999,-0.238183666596899));
#8753=CARTESIAN_POINT('Origin',(0.,-0.04763,0.));
#8754=CARTESIAN_POINT('Origin',(0.,-0.04763,0.));
#8755=CARTESIAN_POINT('Origin',(1.,-0.04763,0.));
#8756=CARTESIAN_POINT('Origin',(1.,0.,0.));
#8757=CARTESIAN_POINT('Origin',(1.,-0.04763,0.));
#8758=CARTESIAN_POINT('Origin',(0.,-0.28578,0.));
#8759=CARTESIAN_POINT('Origin',(0.,-0.04763,0.));
#11214=UNCERTAINTY_MEASURE_WITH_UNIT(LENGTH_MEASURE(0.001),#11259,
'DISTANCE_ACCURACY_VALUE',
'Maximum model space distance between geometric entities at asserted c
onnectivities');
#11228=UNCERTAINTY_MEASURE_WITH_UNIT(LENGTH_MEASURE(0.001),#11259,
'DISTANCE_ACCURACY_VALUE',
'Maximum model space distance between geometric entities at asserted c
onnectivities');
#11244=(
GEOMETRIC_REPRESENTATION_CONTEXT(3)
GLOBAL_UNCERTAINTY_ASSIGNED_CONTEXT((#11214))
GLOBAL_UNIT_ASSIGNED_CONTEXT((#11259,#11261,#11262))
REPRESENTATION_CONTEXT('','3D')
);
#11258=(
GEOMETRIC_REPRESENTATION_CONTEXT(3)
GLOBAL_UNCERTAINTY_ASSIGNED_CONTEXT((#11228))
GLOBAL_UNIT_ASSIGNED_CONTEXT((#11259,#11261,#11262))
REPRESENTATION_CONTEXT('','3D')
);
#11259=(
LENGTH_UNIT()
NAMED_UNIT(*)
SI_UNIT(.CENTI.,.METRE.)
);
#11261=(
NAMED_UNIT(*)
PLANE_ANGLE_UNIT()
SI_UNIT($,.RADIAN.)
);
#11262=(
NAMED_UNIT(*)
SI_UNIT($,.STERADIAN.)
SOLID_ANGLE_UNIT()
);
#11278=SHAPE_DEFINITION_REPRESENTATION(#11307,#11374);
#11307=PRODUCT_DEFINITION_SHAPE('',$,#11404);
#11374=SHAPE_REPRESENTATION('',(#5738),#11244);
#11388=PRODUCT_DEFINITION_CONTEXT('part definition',#11477,'design');
#11404=PRODUCT_DEFINITION('Cage','Cage',#11433,#11388);
#11433=PRODUCT_DEFINITION_FORMATION('',$,#11494);
#11477=APPLICATION_CONTEXT(
'Core Data for Automotive Mechanical Design Process');
#11478=PRODUCT_CONTEXT('part definition',#11477,'mechanical');
#11494=PRODUCT('Cage','Cage','Cage',(#11478));
#11578=COLOUR_RGB('Grey',0.48,0.52,0.57);
#11579=FILL_AREA_STYLE_COLOUR('',#11578);
#11580=FILL_AREA_STYLE('',(#11579));
#11581=SURFACE_STYLE_FILL_AREA(#11580);
#11582=SURFACE_SIDE_STYLE('',(#11581));
#11583=SURFACE_STYLE_USAGE(.BOTH.,#11582);
#11584=PRESENTATION_STYLE_ASSIGNMENT((#11583));
ENDSEC;
END-ISO-10303-21;
